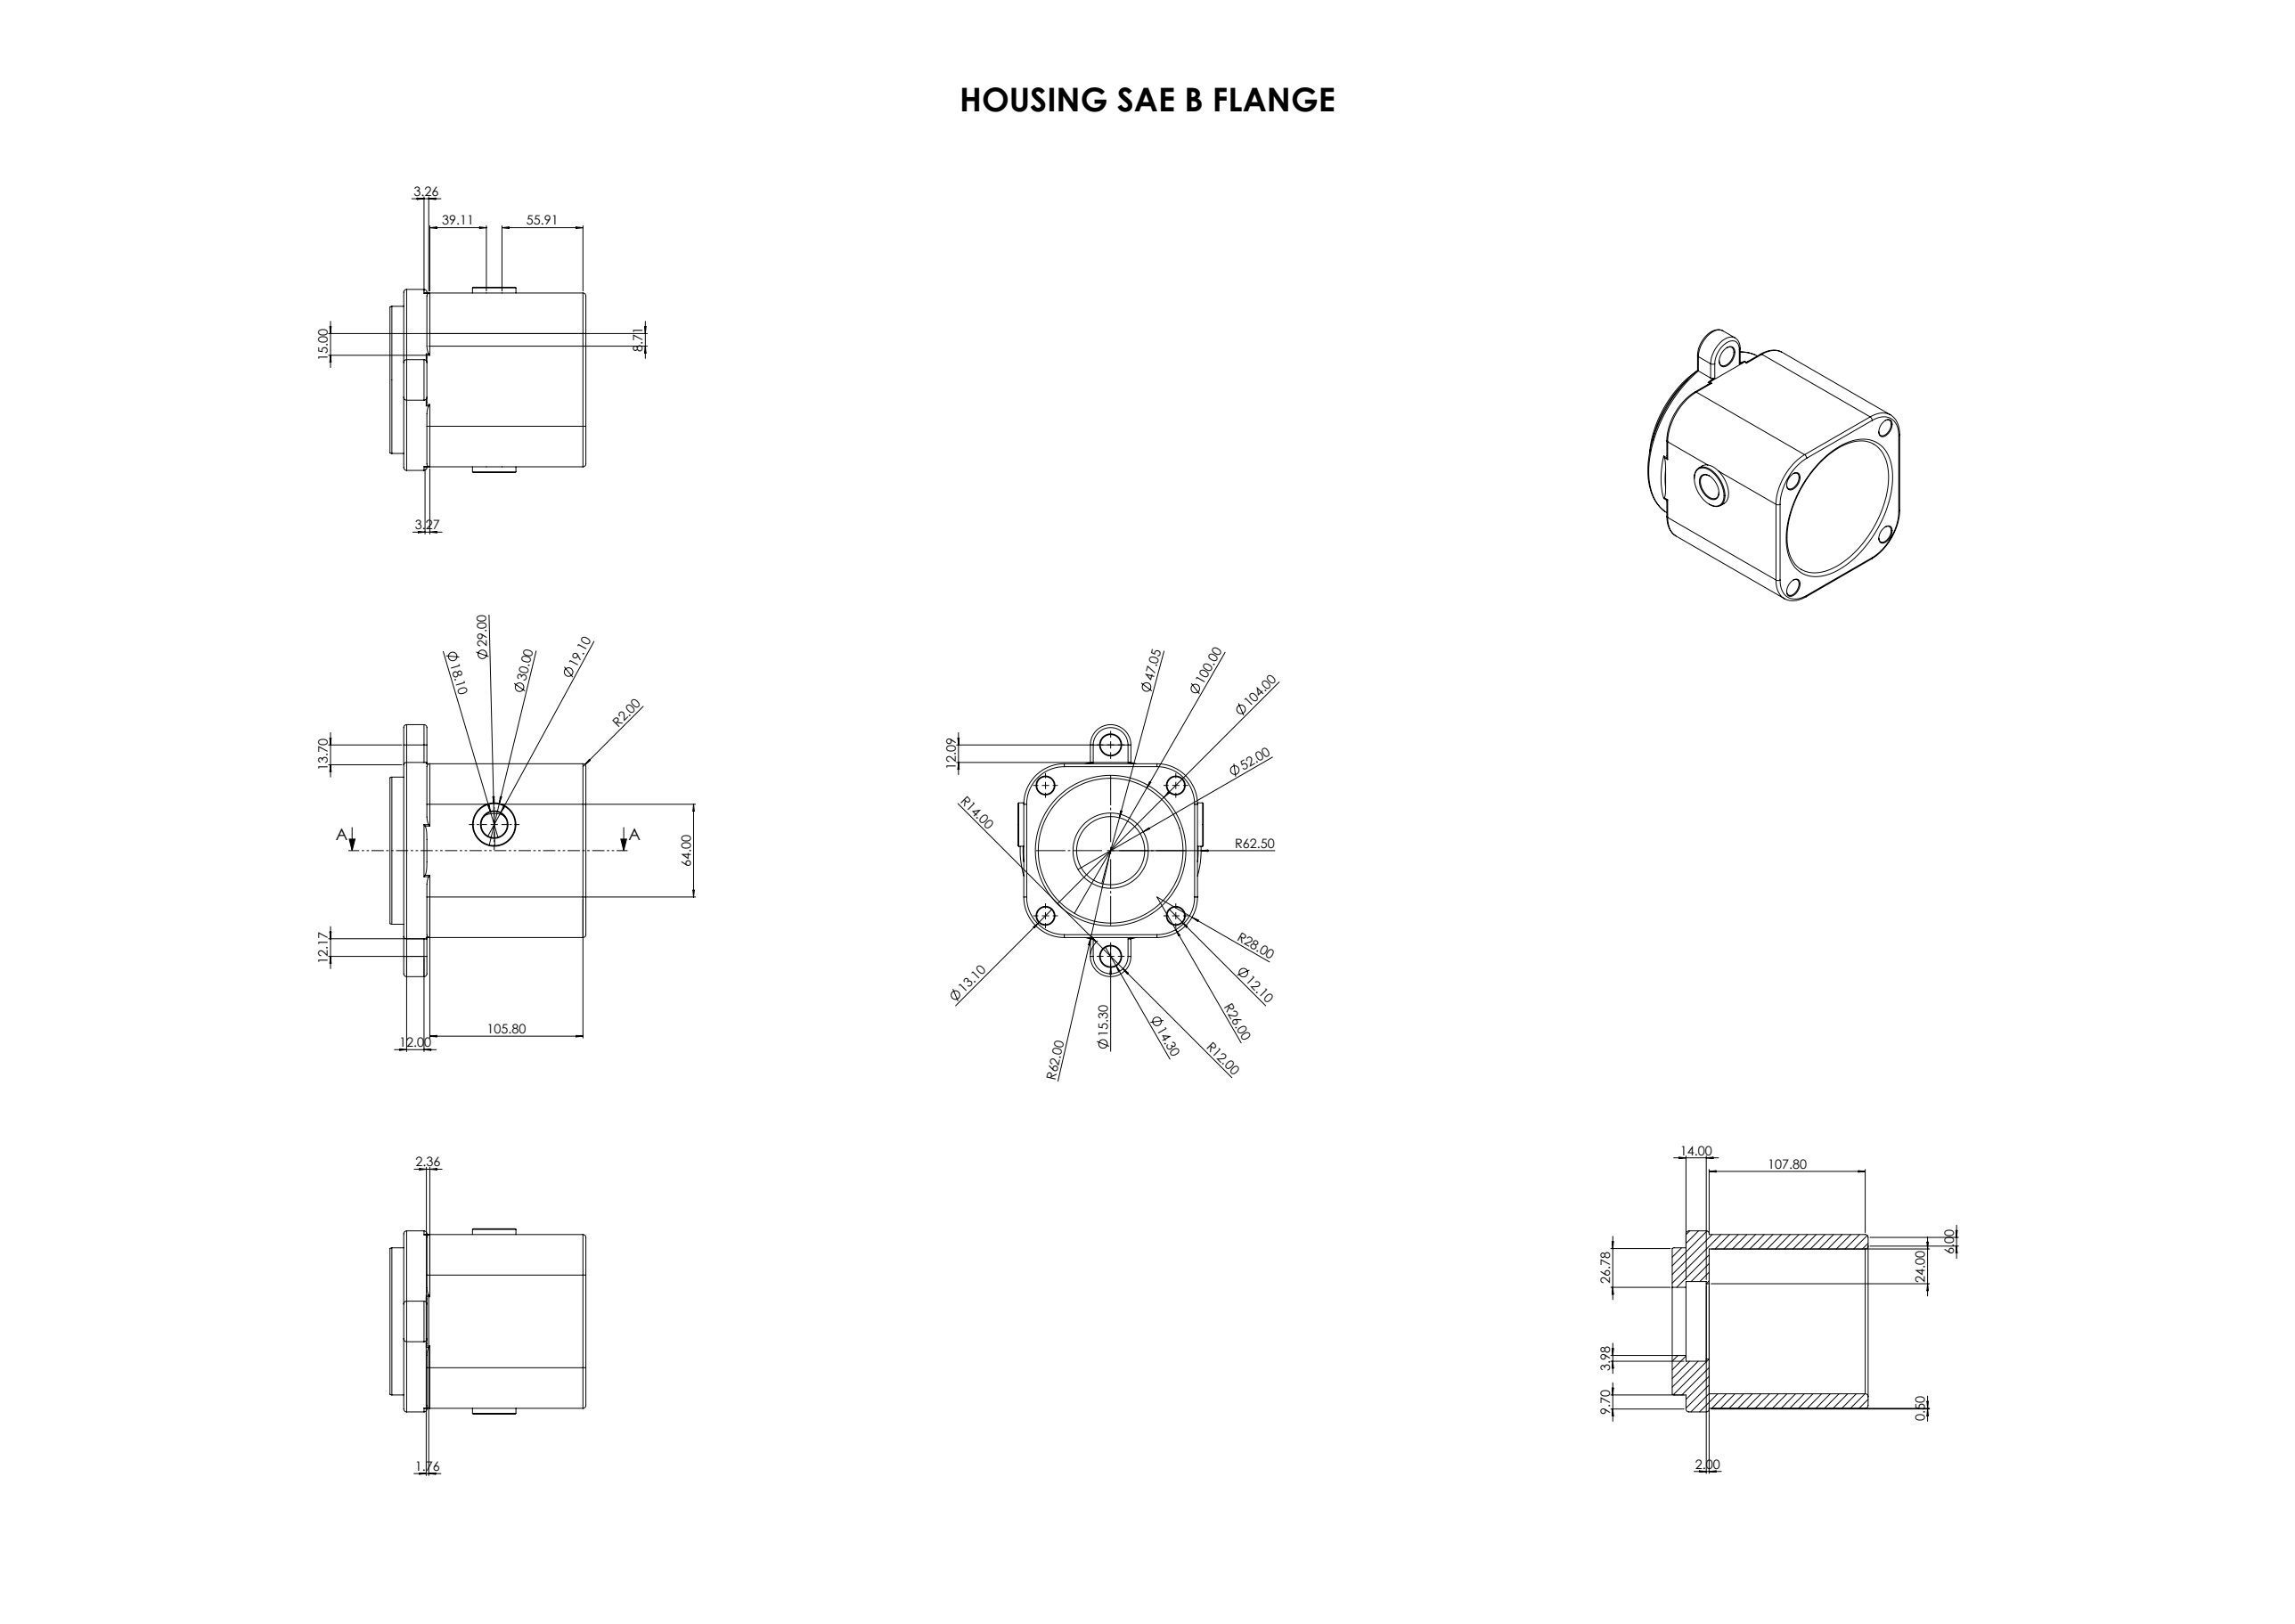
ISO-10303-21;
HEADER;
/* Generated by software containing ST-Developer
 * from STEP Tools, Inc. (www.steptools.com) 
 */

FILE_DESCRIPTION(
/* description */ (''),
/* implementation_level */ '2;1');

FILE_NAME(
/* name */ '01_Housing_SAE_B_Flange.step',
/* time_stamp */ '2026-10-26T07:49:00-07:00',
/* author */ (''),
/* organization */ (''),
/* preprocessor_version */ 'ST-DEVELOPER v20.2',
/* originating_system */ 'Autodesk Translation Framework v15.15.0.0',
/* authorisation */ '');

FILE_SCHEMA (('AUTOMOTIVE_DESIGN { 1 0 10303 214 3 1 1 }'));
ENDSEC;

DATA;
#10=MECHANICAL_DESIGN_GEOMETRIC_PRESENTATION_REPRESENTATION('',(#177),#38507);
#147=SHAPE_REPRESENTATION_RELATIONSHIP('SRR','None',#38575,#162);
#162=ADVANCED_BREP_SHAPE_REPRESENTATION('',(#192),#38492);
#177=STYLED_ITEM('',(#38699),#192);
#192=MANIFOLD_SOLID_BREP('Body1',#15071);
#207=B_SPLINE_SURFACE_WITH_KNOTS('',3,3,((#22067,#22068,#22069,#22070,#22071,
#22072,#22073),(#22074,#22075,#22076,#22077,#22078,#22079,#22080),(#22081,
#22082,#22083,#22084,#22085,#22086,#22087),(#22088,#22089,#22090,#22091,
#22092,#22093,#22094)),.UNSPECIFIED.,.F.,.F.,.F.,(4,4),(4,1,1,1,4),(0.,
1.),(-0.462000333519479,-0.263998422594088,-0.131997148643828,-0.0329961931811326,
4.1253064325321E-6),.UNSPECIFIED.);
#208=B_SPLINE_SURFACE_WITH_KNOTS('',3,3,((#22108,#22109,#22110,#22111,#22112,
#22113,#22114,#22115,#22116,#22117),(#22118,#22119,#22120,#22121,#22122,
#22123,#22124,#22125,#22126,#22127),(#22128,#22129,#22130,#22131,#22132,
#22133,#22134,#22135,#22136,#22137),(#22138,#22139,#22140,#22141,#22142,
#22143,#22144,#22145,#22146,#22147),(#22148,#22149,#22150,#22151,#22152,
#22153,#22154,#22155,#22156,#22157),(#22158,#22159,#22160,#22161,#22162,
#22163,#22164,#22165,#22166,#22167),(#22168,#22169,#22170,#22171,#22172,
#22173,#22174,#22175,#22176,#22177)),.UNSPECIFIED.,.F.,.F.,.F.,(4,1,1,1,
4),(4,1,1,1,1,1,1,4),(0.,0.285714285714286,0.571428571428571,0.785714285714286,
1.),(-7.35549329570849,-7.06046758790365,-6.76544188009881,-6.47041617229397,
-6.17539046448912,-5.88036475668429,-5.58533904887944,-5.2903133410746),
 .UNSPECIFIED.);
#209=B_SPLINE_SURFACE_WITH_KNOTS('',3,3,((#22179,#22180,#22181,#22182,#22183,
#22184,#22185,#22186,#22187,#22188,#22189,#22190,#22191,#22192,#22193,#22194,
#22195,#22196,#22197,#22198,#22199,#22200,#22201,#22202,#22203),(#22204,
#22205,#22206,#22207,#22208,#22209,#22210,#22211,#22212,#22213,#22214,#22215,
#22216,#22217,#22218,#22219,#22220,#22221,#22222,#22223,#22224,#22225,#22226,
#22227,#22228),(#22229,#22230,#22231,#22232,#22233,#22234,#22235,#22236,
#22237,#22238,#22239,#22240,#22241,#22242,#22243,#22244,#22245,#22246,#22247,
#22248,#22249,#22250,#22251,#22252,#22253),(#22254,#22255,#22256,#22257,
#22258,#22259,#22260,#22261,#22262,#22263,#22264,#22265,#22266,#22267,#22268,
#22269,#22270,#22271,#22272,#22273,#22274,#22275,#22276,#22277,#22278),
(#22279,#22280,#22281,#22282,#22283,#22284,#22285,#22286,#22287,#22288,
#22289,#22290,#22291,#22292,#22293,#22294,#22295,#22296,#22297,#22298,#22299,
#22300,#22301,#22302,#22303)),.UNSPECIFIED.,.F.,.F.,.F.,(4,1,4),(4,2,1,
1,1,1,1,1,1,1,1,1,1,1,1,1,1,1,1,1,1,4),(0.,0.571428571428571,1.),(-0.461724827521327,
-0.461389911948815,-0.455622538049454,-0.449855164150094,-0.438320416351374,
-0.415250920753933,-0.392181425156492,-0.369111929559052,-0.346042433961611,
-0.32297293836417,-0.29990344276673,-0.276833947169289,-0.253764451571848,
-0.230694955974407,-0.207625460376967,-0.196090712578246,-0.184555964779526,
-0.138416973584644,-0.115347477987204,-0.0922779823897629,-0.0461389911948815,
0.),.UNSPECIFIED.);
#210=B_SPLINE_SURFACE_WITH_KNOTS('',3,3,((#22314,#22315,#22316,#22317,#22318,
#22319,#22320,#22321,#22322,#22323),(#22324,#22325,#22326,#22327,#22328,
#22329,#22330,#22331,#22332,#22333),(#22334,#22335,#22336,#22337,#22338,
#22339,#22340,#22341,#22342,#22343),(#22344,#22345,#22346,#22347,#22348,
#22349,#22350,#22351,#22352,#22353),(#22354,#22355,#22356,#22357,#22358,
#22359,#22360,#22361,#22362,#22363),(#22364,#22365,#22366,#22367,#22368,
#22369,#22370,#22371,#22372,#22373)),.UNSPECIFIED.,.F.,.F.,.F.,(4,1,1,4),
(4,1,1,1,1,1,1,4),(0.,0.285714285714286,0.571428571428571,1.),(4.72327004783361,
5.43406096940559,6.14485189097757,6.85564281254955,7.56643373412153,8.27722465569351,
8.98801557726548,9.69880649883746),.UNSPECIFIED.);
#211=B_SPLINE_SURFACE_WITH_KNOTS('',3,3,((#22374,#22375,#22376,#22377,#22378,
#22379),(#22380,#22381,#22382,#22383,#22384,#22385),(#22386,#22387,#22388,
#22389,#22390,#22391),(#22392,#22393,#22394,#22395,#22396,#22397)),
 .UNSPECIFIED.,.F.,.F.,.F.,(4,4),(4,1,1,4),(0.,1.),(-0.461769339103211,
-0.197899101291517,-0.0659639823856703,3.57706725334641E-6),
 .UNSPECIFIED.);
#212=B_SPLINE_SURFACE_WITH_KNOTS('',3,3,((#22412,#22413,#22414,#22415,#22416,
#22417,#22418,#22419,#22420,#22421),(#22422,#22423,#22424,#22425,#22426,
#22427,#22428,#22429,#22430,#22431),(#22432,#22433,#22434,#22435,#22436,
#22437,#22438,#22439,#22440,#22441),(#22442,#22443,#22444,#22445,#22446,
#22447,#22448,#22449,#22450,#22451),(#22452,#22453,#22454,#22455,#22456,
#22457,#22458,#22459,#22460,#22461),(#22462,#22463,#22464,#22465,#22466,
#22467,#22468,#22469,#22470,#22471),(#22472,#22473,#22474,#22475,#22476,
#22477,#22478,#22479,#22480,#22481)),.UNSPECIFIED.,.F.,.F.,.F.,(4,1,1,1,
4),(4,1,1,1,1,1,1,4),(0.,0.285714285714286,0.571428571428571,0.785714285714286,
1.),(-7.35549329570849,-7.06046758790365,-6.76544188009881,-6.47041617229397,
-6.17539046448913,-5.88036475668429,-5.58533904887945,-5.29031334107461),
 .UNSPECIFIED.);
#213=B_SPLINE_SURFACE_WITH_KNOTS('',3,3,((#22485,#22486,#22487,#22488,#22489,
#22490),(#22491,#22492,#22493,#22494,#22495,#22496),(#22497,#22498,#22499,
#22500,#22501,#22502),(#22503,#22504,#22505,#22506,#22507,#22508)),
 .UNSPECIFIED.,.F.,.F.,.F.,(4,4),(4,1,1,4),(0.,1.),(-0.461725499841195,
-0.395764714149595,-0.263843142766397,0.),.UNSPECIFIED.);
#214=B_SPLINE_SURFACE_WITH_KNOTS('',3,3,((#22519,#22520,#22521,#22522,#22523,
#22524,#22525,#22526,#22527,#22528),(#22529,#22530,#22531,#22532,#22533,
#22534,#22535,#22536,#22537,#22538),(#22539,#22540,#22541,#22542,#22543,
#22544,#22545,#22546,#22547,#22548),(#22549,#22550,#22551,#22552,#22553,
#22554,#22555,#22556,#22557,#22558),(#22559,#22560,#22561,#22562,#22563,
#22564,#22565,#22566,#22567,#22568),(#22569,#22570,#22571,#22572,#22573,
#22574,#22575,#22576,#22577,#22578)),.UNSPECIFIED.,.F.,.F.,.F.,(4,1,1,4),
(4,1,1,1,1,1,1,4),(0.,0.285714285714286,0.571428571428571,1.),(4.72327004804774,
5.43406096961972,6.1448518911917,6.85564281276368,7.56643373433566,8.27722465590764,
8.98801557747962,9.6988064990516),.UNSPECIFIED.);
#256=TOROIDAL_SURFACE('',#15366,60.5,2.);
#257=TOROIDAL_SURFACE('',#15369,12.,2.);
#258=TOROIDAL_SURFACE('',#15373,60.5,2.);
#259=TOROIDAL_SURFACE('',#15374,12.,2.);
#260=TOROIDAL_SURFACE('',#15383,60.5,2.);
#261=TOROIDAL_SURFACE('',#15387,12.,2.);
#262=TOROIDAL_SURFACE('',#15394,60.5,2.);
#263=TOROIDAL_SURFACE('',#15398,12.,2.);
#264=TOROIDAL_SURFACE('',#15402,48.8,2.);
#265=TOROIDAL_SURFACE('',#15409,26.,2.);
#266=TOROIDAL_SURFACE('',#15415,26.,2.);
#267=TOROIDAL_SURFACE('',#15425,26.,2.);
#268=TOROIDAL_SURFACE('',#15433,26.,2.);
#269=TOROIDAL_SURFACE('',#15442,26.,2.);
#270=TOROIDAL_SURFACE('',#15447,26.,2.);
#271=TOROIDAL_SURFACE('',#15452,26.,2.);
#272=TOROIDAL_SURFACE('',#15457,26.,2.);
#273=TOROIDAL_SURFACE('',#15461,52.,2.);
#293=ELLIPSE('',#15321,13.946906437048,2.);
#294=ELLIPSE('',#15324,13.946906437048,2.);
#295=ELLIPSE('',#15327,13.946906437048,2.);
#296=ELLIPSE('',#15331,13.946906437048,2.);
#297=ELLIPSE('',#15340,13.946906437048,2.);
#298=ELLIPSE('',#15343,13.946906437048,2.);
#299=ELLIPSE('',#15346,13.946906437048,2.);
#300=ELLIPSE('',#15350,13.946906437048,2.);
#332=(
BOUNDED_CURVE()
B_SPLINE_CURVE(2,(#21090,#21091,#21092),.UNSPECIFIED.,.F.,.F.)
B_SPLINE_CURVE_WITH_KNOTS((3,3),(-9.16934047811363,-8.99429341935052),
 .UNSPECIFIED.)
CURVE()
GEOMETRIC_REPRESENTATION_ITEM()
RATIONAL_B_SPLINE_CURVE((1.20544110146931,1.20730170334354,1.20901639344262))
REPRESENTATION_ITEM('')
);
#333=(
BOUNDED_CURVE()
B_SPLINE_CURVE(2,(#21112,#21113,#21114),.UNSPECIFIED.,.F.,.F.)
B_SPLINE_CURVE_WITH_KNOTS((3,3),(-4.88014350616112,-4.705096447398),
 .UNSPECIFIED.)
CURVE()
GEOMETRIC_REPRESENTATION_ITEM()
RATIONAL_B_SPLINE_CURVE((1.20901639344263,1.20730170334354,1.20544110146931))
REPRESENTATION_ITEM('')
);
#334=(
BOUNDED_CURVE()
B_SPLINE_CURVE(2,(#21198,#21199,#21200),.UNSPECIFIED.,.F.,.F.)
B_SPLINE_CURVE_WITH_KNOTS((3,3),(-4.88014350616107,-4.70509644739795),
 .UNSPECIFIED.)
CURVE()
GEOMETRIC_REPRESENTATION_ITEM()
RATIONAL_B_SPLINE_CURVE((1.20901639344262,1.20730170334354,1.20544110146931))
REPRESENTATION_ITEM('')
);
#335=(
BOUNDED_CURVE()
B_SPLINE_CURVE(2,(#21291,#21292,#21293),.UNSPECIFIED.,.F.,.F.)
B_SPLINE_CURVE_WITH_KNOTS((3,3),(-9.16934047811369,-8.99429341935056),
 .UNSPECIFIED.)
CURVE()
GEOMETRIC_REPRESENTATION_ITEM()
RATIONAL_B_SPLINE_CURVE((1.20544110146931,1.20730170334354,1.20901639344263))
REPRESENTATION_ITEM('')
);
#417=FACE_BOUND('',#2507,.T.);
#418=FACE_BOUND('',#2510,.T.);
#419=FACE_BOUND('',#2514,.T.);
#420=FACE_BOUND('',#2518,.T.);
#421=FACE_BOUND('',#2524,.T.);
#422=FACE_BOUND('',#2525,.T.);
#423=FACE_BOUND('',#2526,.T.);
#424=FACE_BOUND('',#2527,.T.);
#425=FACE_BOUND('',#2528,.T.);
#426=FACE_BOUND('',#2556,.T.);
#427=FACE_BOUND('',#2557,.T.);
#428=FACE_BOUND('',#2558,.T.);
#429=FACE_BOUND('',#2612,.T.);
#430=FACE_BOUND('',#2613,.T.);
#431=FACE_BOUND('',#2629,.T.);
#432=FACE_BOUND('',#2632,.T.);
#433=FACE_BOUND('',#2635,.T.);
#434=FACE_BOUND('',#2637,.T.);
#558=PLANE('',#15260);
#559=PLANE('',#15265);
#560=PLANE('',#15274);
#561=PLANE('',#15282);
#562=PLANE('',#15295);
#563=PLANE('',#15320);
#564=PLANE('',#15322);
#565=PLANE('',#15323);
#566=PLANE('',#15325);
#567=PLANE('',#15326);
#568=PLANE('',#15330);
#569=PLANE('',#15339);
#570=PLANE('',#15341);
#571=PLANE('',#15342);
#572=PLANE('',#15344);
#573=PLANE('',#15345);
#574=PLANE('',#15349);
#575=PLANE('',#15358);
#576=PLANE('',#15382);
#577=PLANE('',#15391);
#578=PLANE('',#15393);
#579=PLANE('',#15401);
#580=PLANE('',#15414);
#581=PLANE('',#15422);
#582=PLANE('',#15430);
#583=PLANE('',#15438);
#584=PLANE('',#15473);
#585=PLANE('',#15474);
#586=PLANE('',#15475);
#587=PLANE('',#15476);
#588=PLANE('',#15480);
#589=PLANE('',#15484);
#590=PLANE('',#15488);
#591=PLANE('',#15489);
#592=PLANE('',#15492);
#593=PLANE('',#15493);
#1009=B_SPLINE_CURVE_WITH_KNOTS('',3,(#20904,#20905,#20906,#20907,#20908,
#20909,#20910,#20911,#20912,#20913),.UNSPECIFIED.,.F.,.F.,(4,2,2,2,4),(3.93196561503714,
3.98793494995107,4.45544073881652,4.92294652768197,4.9789158625959),
 .UNSPECIFIED.);
#1010=B_SPLINE_CURVE_WITH_KNOTS('',3,(#20956,#20957,#20958,#20959,#20960,
#20961,#20962,#20963,#20964,#20965),.UNSPECIFIED.,.F.,.F.,(4,2,2,2,4),(3.93196561503714,
3.98793494995108,4.45544073881652,4.92294652768197,4.97891586259591),
 .UNSPECIFIED.);
#1011=B_SPLINE_CURVE_WITH_KNOTS('',3,(#20998,#20999,#21000,#21001,#21002),
 .UNSPECIFIED.,.F.,.F.,(4,1,4),(4.72327004821084,5.43406096940559,5.4438775737049),
 .UNSPECIFIED.);
#1012=B_SPLINE_CURVE_WITH_KNOTS('',3,(#21005,#21006,#21007,#21008,#21009,
#21010,#21011,#21012,#21013),.UNSPECIFIED.,.F.,.F.,(4,1,1,1,1,1,4),(5.4438775737049,
6.14485189097757,6.85564281254955,7.56643373412153,8.27722465569351,8.98801557726548,
9.69880649883746),.UNSPECIFIED.);
#1013=B_SPLINE_CURVE_WITH_KNOTS('',3,(#21075,#21076,#21077,#21078,#21079,
#21080,#21081,#21082),.UNSPECIFIED.,.F.,.F.,(4,2,2,4),(0.909514729117648,
0.949358494570548,1.0210248366573,1.05494162626089),.UNSPECIFIED.);
#1014=B_SPLINE_CURVE_WITH_KNOTS('',3,(#21086,#21087,#21088,#21089),
 .UNSPECIFIED.,.F.,.F.,(4,4),(-0.0999299837778113,0.),.UNSPECIFIED.);
#1015=B_SPLINE_CURVE_WITH_KNOTS('',3,(#21118,#21119,#21120,#21121,#21122,
#21123,#21124,#21125,#21126,#21127),.UNSPECIFIED.,.F.,.F.,(4,2,2,2,4),(2.62788407869953,
2.67944373713314,2.73012587368336,2.74303185768817,2.7532959630073),
 .UNSPECIFIED.);
#1016=B_SPLINE_CURVE_WITH_KNOTS('',3,(#21137,#21138,#21139,#21140,#21141,
#21142,#21143,#21144,#21145,#21146),.UNSPECIFIED.,.F.,.F.,(4,2,2,2,4),(1.79948460602208,
1.8527312039325,2.06373263634258,2.27473406875267,2.69673693357283),
 .UNSPECIFIED.);
#1017=B_SPLINE_CURVE_WITH_KNOTS('',3,(#21150,#21151,#21152,#21153,#21154,
#21155,#21156,#21157,#21158,#21159),.UNSPECIFIED.,.F.,.F.,(4,2,2,2,4),(4.15220051801173,
4.5742033828319,4.78520481524198,4.99620624765207,5.04945284556248),
 .UNSPECIFIED.);
#1018=B_SPLINE_CURVE_WITH_KNOTS('',3,(#21174,#21175,#21176,#21177,#21178,
#21179,#21180,#21181,#21182,#21183),.UNSPECIFIED.,.F.,.F.,(4,2,2,2,4),(0.917765321002435,
0.928029426321564,0.940935410326375,0.991617546876601,1.04317720531021),
 .UNSPECIFIED.);
#1019=B_SPLINE_CURVE_WITH_KNOTS('',3,(#21189,#21190,#21191,#21192,#21193,
#21194,#21195,#21196),.UNSPECIFIED.,.F.,.F.,(4,2,2,4),(0.423927454431935,
0.457844244035524,0.529510586122272,0.569354351575173),.UNSPECIFIED.);
#1020=B_SPLINE_CURVE_WITH_KNOTS('',3,(#21201,#21202,#21203,#21204),
 .UNSPECIFIED.,.F.,.F.,(4,4),(-0.0999299524181728,0.),.UNSPECIFIED.);
#1021=B_SPLINE_CURVE_WITH_KNOTS('',3,(#21213,#21214,#21215,#21216,#21217,
#21218,#21219,#21220),.UNSPECIFIED.,.F.,.F.,(4,2,2,4),(0.444478348171076,
0.457897885991393,0.533188282866212,0.608478679741031),.UNSPECIFIED.);
#1022=B_SPLINE_CURVE_WITH_KNOTS('',3,(#21227,#21228,#21229,#21230,#21231,
#21232,#21233,#21234),.UNSPECIFIED.,.F.,.F.,(4,2,2,4),(0.608478679741031,
0.68376907661585,0.759059473490669,0.772479011310987),.UNSPECIFIED.);
#1023=B_SPLINE_CURVE_WITH_KNOTS('',3,(#21236,#21237,#21238,#21239,#21240,
#21241,#21242,#21243),.UNSPECIFIED.,.F.,.F.,(4,2,2,4),(1.27628724021533,
1.34251720334849,1.43059045082634,1.8254794159769),.UNSPECIFIED.);
#1024=B_SPLINE_CURVE_WITH_KNOTS('',3,(#21246,#21247,#21248,#21249,#21250,
#21251,#21252,#21253),.UNSPECIFIED.,.F.,.F.,(4,2,2,4),(0.537818085774576,
0.932707050925141,1.02078029840299,1.08701026153615),.UNSPECIFIED.);
#1025=B_SPLINE_CURVE_WITH_KNOTS('',3,(#21256,#21257,#21258,#21259,#21260,
#21261,#21262,#21263),.UNSPECIFIED.,.F.,.F.,(4,2,2,4),(1.27628724021533,
1.34251720334849,1.43059045082634,1.8254794159769),.UNSPECIFIED.);
#1026=B_SPLINE_CURVE_WITH_KNOTS('',3,(#21266,#21267,#21268,#21269,#21270,
#21271,#21272,#21273),.UNSPECIFIED.,.F.,.F.,(4,2,2,4),(0.537818085774576,
0.932707050925141,1.02078029840299,1.08701026153615),.UNSPECIFIED.);
#1027=B_SPLINE_CURVE_WITH_KNOTS('',3,(#21276,#21277,#21278,#21279,#21280,
#21281,#21282,#21283),.UNSPECIFIED.,.F.,.F.,(4,2,2,4),(0.909514729117652,
0.949358494570554,1.0210248366573,1.05494162626089),.UNSPECIFIED.);
#1028=B_SPLINE_CURVE_WITH_KNOTS('',3,(#21287,#21288,#21289,#21290),
 .UNSPECIFIED.,.F.,.F.,(4,4),(-0.099929983777859,0.),.UNSPECIFIED.);
#1029=B_SPLINE_CURVE_WITH_KNOTS('',3,(#21313,#21314,#21315,#21316,#21317,
#21318,#21319,#21320,#21321,#21322),.UNSPECIFIED.,.F.,.F.,(4,2,2,2,4),(2.62788407869953,
2.67944373713314,2.73012587368336,2.74303185768817,2.7532959630073),
 .UNSPECIFIED.);
#1030=B_SPLINE_CURVE_WITH_KNOTS('',3,(#21332,#21333,#21334,#21335,#21336,
#21337,#21338,#21339,#21340,#21341),.UNSPECIFIED.,.F.,.F.,(4,2,2,2,4),(1.79948460602208,
1.8527312039325,2.06373263634258,2.27473406875267,2.69673693357283),
 .UNSPECIFIED.);
#1031=B_SPLINE_CURVE_WITH_KNOTS('',3,(#21345,#21346,#21347,#21348,#21349,
#21350,#21351,#21352,#21353,#21354),.UNSPECIFIED.,.F.,.F.,(4,2,2,2,4),(4.15220051801173,
4.5742033828319,4.78520481524198,4.99620624765207,5.04945284556248),
 .UNSPECIFIED.);
#1032=B_SPLINE_CURVE_WITH_KNOTS('',3,(#21369,#21370,#21371,#21372,#21373,
#21374,#21375,#21376,#21377,#21378),.UNSPECIFIED.,.F.,.F.,(4,2,2,2,4),(0.917765321002435,
0.928029426321564,0.940935410326375,0.991617546876601,1.04317720531021),
 .UNSPECIFIED.);
#1033=B_SPLINE_CURVE_WITH_KNOTS('',3,(#21384,#21385,#21386,#21387,#21388,
#21389,#21390,#21391),.UNSPECIFIED.,.F.,.F.,(4,2,2,4),(0.42392745443194,
0.457844244035527,0.529510586122276,0.569354351575178),.UNSPECIFIED.);
#1034=B_SPLINE_CURVE_WITH_KNOTS('',3,(#21392,#21393,#21394,#21395),
 .UNSPECIFIED.,.F.,.F.,(4,4),(-0.0999299524180764,0.),.UNSPECIFIED.);
#1035=B_SPLINE_CURVE_WITH_KNOTS('',3,(#21402,#21403,#21404,#21405,#21406,
#21407,#21408,#21409),.UNSPECIFIED.,.F.,.F.,(4,2,2,4),(0.444478348171076,
0.457897885991393,0.533188282866212,0.608478679741031),.UNSPECIFIED.);
#1036=B_SPLINE_CURVE_WITH_KNOTS('',3,(#21416,#21417,#21418,#21419,#21420,
#21421,#21422,#21423),.UNSPECIFIED.,.F.,.F.,(4,2,2,4),(0.608478679741031,
0.68376907661585,0.759059473490669,0.772479011310987),.UNSPECIFIED.);
#1037=B_SPLINE_CURVE_WITH_KNOTS('',3,(#21425,#21426,#21427,#21428,#21429,
#21430,#21431,#21432),.UNSPECIFIED.,.F.,.F.,(4,2,2,4),(1.27628724021533,
1.34251720334849,1.43059045082634,1.8254794159769),.UNSPECIFIED.);
#1038=B_SPLINE_CURVE_WITH_KNOTS('',3,(#21435,#21436,#21437,#21438,#21439,
#21440,#21441,#21442),.UNSPECIFIED.,.F.,.F.,(4,2,2,4),(0.537818085774576,
0.932707050925141,1.02078029840299,1.08701026153615),.UNSPECIFIED.);
#1039=B_SPLINE_CURVE_WITH_KNOTS('',3,(#21445,#21446,#21447,#21448,#21449,
#21450,#21451,#21452),.UNSPECIFIED.,.F.,.F.,(4,2,2,4),(1.27628724021533,
1.34251720334849,1.43059045082634,1.8254794159769),.UNSPECIFIED.);
#1040=B_SPLINE_CURVE_WITH_KNOTS('',3,(#21455,#21456,#21457,#21458,#21459,
#21460,#21461,#21462),.UNSPECIFIED.,.F.,.F.,(4,2,2,4),(0.537818085774576,
0.932707050925141,1.02078029840299,1.08701026153615),.UNSPECIFIED.);
#1041=B_SPLINE_CURVE_WITH_KNOTS('',3,(#21491,#21492,#21493,#21494,#21495,
#21496,#21497,#21498,#21499,#21500,#21501,#21502,#21503,#21504),
 .UNSPECIFIED.,.F.,.F.,(4,2,2,2,2,2,4),(-0.0007960460749726,0.,0.0734612670102269,
0.144831741121295,0.230214082122091,0.299049896049864,0.361337990313849),
 .UNSPECIFIED.);
#1042=B_SPLINE_CURVE_WITH_KNOTS('',3,(#21505,#21506,#21507,#21508,#21509,
#21510,#21511,#21512,#21513,#21514,#21515,#21516,#21517,#21518),
 .UNSPECIFIED.,.F.,.F.,(4,2,2,2,2,2,4),(-0.723464285927595,-0.722647521542398,
-0.649394023974264,-0.578539147977434,-0.492689132311904,-0.42364974758642,
-0.361323760770171),.UNSPECIFIED.);
#1043=B_SPLINE_CURVE_WITH_KNOTS('',3,(#21528,#21529,#21530,#21531,#21532,
#21533,#21534,#21535,#21536,#21537,#21538,#21539,#21540,#21541),
 .UNSPECIFIED.,.F.,.F.,(4,2,2,2,2,2,4),(-0.361281373349619,-0.299845297677646,
-0.234790847494551,-0.156277186792366,-0.0770809532846638,0.,0.000773217160646022),
 .UNSPECIFIED.);
#1044=B_SPLINE_CURVE_WITH_KNOTS('',3,(#21544,#21545,#21546,#21547,#21548,
#21549,#21550,#21551,#21552,#21553,#21554,#21555,#21556,#21557),
 .UNSPECIFIED.,.F.,.F.,(4,2,2,2,2,2,4),(-0.723464285923361,-0.722647521538168,
-0.649394023970219,-0.578539147973825,-0.492689132308839,-0.423649747583786,
-0.361323760767944),.UNSPECIFIED.);
#1045=B_SPLINE_CURVE_WITH_KNOTS('',3,(#21692,#21693,#21694,#21695,#21696,
#21697,#21698,#21699,#21700,#21701,#21702,#21703,#21704,#21705,#21706,#21707,
#21708,#21709,#21710,#21711,#21712,#21713,#21714,#21715,#21716),
 .UNSPECIFIED.,.F.,.F.,(4,1,1,1,1,1,1,1,1,1,1,1,1,1,1,1,1,1,1,1,2,4),(0.,
0.0461389911948815,0.0922779823897629,0.115347477987204,0.138416973584644,
0.184555964779526,0.196090712578246,0.207625460376967,0.230694955974407,
0.253764451571848,0.276833947169289,0.29990344276673,0.32297293836417,0.346042433961611,
0.369111929559052,0.392181425156492,0.415250920753933,0.438320416351374,
0.449855164150094,0.455622538049454,0.461389911948815,0.46172446147336),
 .UNSPECIFIED.);
#1046=B_SPLINE_CURVE_WITH_KNOTS('',3,(#21718,#21719,#21720,#21721,#21722,
#21723,#21724,#21725,#21726,#21727),.UNSPECIFIED.,.F.,.F.,(4,1,1,1,1,1,
1,4),(5.2903133410746,5.58533904887944,5.88036475668429,6.17539046448912,
6.47041617229397,6.76544188009881,7.06046758790365,7.35549329570849),
 .UNSPECIFIED.);
#1047=B_SPLINE_CURVE_WITH_KNOTS('',3,(#21729,#21730,#21731,#21732,#21733,
#21734,#21735),.UNSPECIFIED.,.F.,.F.,(4,1,1,1,4),(-4.1253064325321E-6,0.0329961931811326,
0.131997148643828,0.263998422594088,0.462000333519479),.UNSPECIFIED.);
#1048=B_SPLINE_CURVE_WITH_KNOTS('',3,(#21736,#21737,#21738,#21739,#21740,
#21741,#21742,#21743,#21744,#21745,#21746,#21747,#21748,#21749,#21750,#21751,
#21752,#21753,#21754,#21755,#21756,#21757,#21758,#21759,#21760,#21761,#21762,
#21763,#21764,#21765,#21766,#21767,#21768,#21769,#21770,#21771,#21772,#21773,
#21774,#21775,#21776,#21777,#21778,#21779,#21780,#21781,#21782,#21783,#21784,
#21785,#21786,#21787,#21788,#21789,#21790,#21791,#21792,#21793,#21794,#21795,
#21796,#21797,#21798,#21799,#21800,#21801,#21802,#21803,#21804,#21805,#21806,
#21807,#21808,#21809,#21810,#21811,#21812,#21813,#21814,#21815,#21816,#21817,
#21818,#21819,#21820,#21821,#21822,#21823,#21824,#21825,#21826,#21827,#21828,
#21829,#21830,#21831,#21832,#21833,#21834,#21835,#21836,#21837,#21838,#21839,
#21840,#21841,#21842,#21843,#21844,#21845,#21846,#21847,#21848,#21849,#21850,
#21851,#21852,#21853,#21854,#21855,#21856,#21857,#21858,#21859,#21860,#21861,
#21862,#21863,#21864,#21865,#21866,#21867,#21868,#21869,#21870,#21871,#21872,
#21873,#21874,#21875,#21876,#21877,#21878,#21879,#21880,#21881,#21882,#21883,
#21884,#21885,#21886,#21887,#21888,#21889),.UNSPECIFIED.,.F.,.F.,(4,3,3,
3,3,3,3,3,3,3,3,3,3,3,3,3,3,3,3,3,3,3,3,3,3,3,3,3,3,3,3,3,3,3,3,3,3,3,3,
3,3,3,3,3,3,3,3,3,3,3,3,4),(-9.23633566839803,-9.12960054610899,-9.02995313475932,
-8.98820092273608,-8.94767164911647,-8.85551547280586,-8.76973813956101,
-8.76335929649525,-8.67204037852948,-8.58170123880419,-8.50986230805487,
-8.41197083977331,-8.31595106965646,-8.27742304064402,-8.18141772850045,
-8.08522998019979,-8.07506594002406,-7.96624383986804,-7.85665330525787,
-7.74811076545733,-7.64783984054416,-7.56639692453424,-7.46050702505756,
-7.35408928718672,-7.24751062386446,-7.21105298394138,-7.11797817184964,
-7.02480289993274,-6.98739369316414,-6.87981578778465,-6.85563657893624,
-6.75528006343046,-6.64913220023725,-6.54164653415872,-6.43390512945243,
-6.37349276133023,-6.27658287658477,-6.1795448081392,-6.14462846979886,
-6.04725880022175,-5.9475667529657,-5.93469080516676,-5.83694309104053,
-5.73794849627641,-5.67251567403569,-5.57655253596878,-5.48609949444031,
-5.43374272495868,-5.34284104121183,-5.3056567205391,-5.19777701987056,
-5.18574149361684),.UNSPECIFIED.);
#1049=B_SPLINE_CURVE_WITH_KNOTS('',3,(#21892,#21893,#21894,#21895,#21896,
#21897),.UNSPECIFIED.,.F.,.F.,(4,1,1,4),(0.,0.263843142766397,0.395764714149595,
0.461725499841195),.UNSPECIFIED.);
#1050=B_SPLINE_CURVE_WITH_KNOTS('',3,(#21899,#21900,#21901,#21902,#21903,
#21904,#21905,#21906,#21907,#21908),.UNSPECIFIED.,.F.,.F.,(4,1,1,1,1,1,
1,4),(5.29031334107461,5.58533904887945,5.88036475668429,6.17539046448913,
6.47041617229397,6.76544188009881,7.06046758790365,7.35549329570849),
 .UNSPECIFIED.);
#1051=B_SPLINE_CURVE_WITH_KNOTS('',3,(#21910,#21911,#21912,#21913,#21914,
#21915),.UNSPECIFIED.,.F.,.F.,(4,1,1,4),(-3.57706725334641E-6,0.0659639823856703,
0.197899101291517,0.461769339103211),.UNSPECIFIED.);
#1052=B_SPLINE_CURVE_WITH_KNOTS('',3,(#21916,#21917,#21918,#21919,#21920,
#21921,#21922,#21923,#21924,#21925,#21926,#21927,#21928,#21929,#21930,#21931,
#21932,#21933,#21934,#21935,#21936,#21937,#21938,#21939,#21940,#21941,#21942,
#21943,#21944,#21945,#21946,#21947,#21948,#21949,#21950,#21951,#21952,#21953,
#21954,#21955,#21956,#21957,#21958,#21959,#21960,#21961,#21962,#21963,#21964,
#21965,#21966,#21967,#21968,#21969,#21970,#21971,#21972,#21973,#21974,#21975,
#21976,#21977,#21978,#21979,#21980,#21981,#21982,#21983,#21984,#21985,#21986,
#21987,#21988,#21989,#21990,#21991,#21992,#21993,#21994,#21995,#21996,#21997,
#21998,#21999,#22000,#22001,#22002,#22003,#22004,#22005,#22006,#22007,#22008,
#22009,#22010,#22011,#22012,#22013,#22014,#22015,#22016,#22017,#22018,#22019,
#22020,#22021,#22022,#22023,#22024,#22025,#22026,#22027,#22028,#22029,#22030,
#22031,#22032,#22033,#22034,#22035,#22036,#22037,#22038,#22039,#22040,#22041,
#22042,#22043,#22044,#22045,#22046,#22047,#22048,#22049,#22050,#22051,#22052,
#22053,#22054,#22055,#22056,#22057,#22058,#22059,#22060,#22061,#22062,#22063,
#22064,#22065,#22066),.UNSPECIFIED.,.F.,.F.,(4,3,3,3,3,3,3,3,3,3,3,3,3,
3,3,3,3,3,3,3,3,3,3,3,3,3,3,3,3,3,3,3,3,3,3,3,3,3,3,3,3,3,3,3,3,3,3,3,3,
3,4),(-9.23633566861216,-9.12960054616757,-9.0301001347754,-8.98819964439314,
-8.9476716491939,-8.85551547287179,-8.77004832787379,-8.76335929654967,
-8.67183742403758,-8.58130233357639,-8.50986230801197,-8.41188984789292,
-8.31575746142269,-8.277426795238,-8.17624636762553,-8.07506594001306,-7.96541085300417,
-7.85497781952315,-7.74563908368099,-7.64783984052849,-7.56643652217298,
-7.46139284189079,-7.35584564549624,-7.25012317373638,-7.21105298394139,
-7.1181354465781,-7.02511356178625,-6.98739369309937,-6.88169773695743,
-6.85571344061752,-6.75528006328435,-6.64904197167172,-6.54161818053077,
-6.43368025611171,-6.37349276120329,-6.27597952064751,-6.17860698749197,
-6.14486393337072,-6.04674431800307,-5.94656644708164,-5.93469080503813,
-5.83307322116587,-5.7296525497896,-5.67251567404192,-5.56269437350081,
-5.48609949447997,-5.43365613366603,-5.33247743921033,-5.30565672055846,
-5.20312542921902,-5.18574149383096),.UNSPECIFIED.);
#1053=B_SPLINE_CURVE_WITH_KNOTS('',3,(#22096,#22097,#22098,#22099,#22100,
#22101,#22102,#22103,#22104,#22105,#22106,#22107),.UNSPECIFIED.,.F.,.F.,
(4,2,2,2,2,4),(0.,0.374578330850399,0.631956342435387,0.751788955793774,
0.804327350058264,0.853099247911436),.UNSPECIFIED.);
#1054=B_SPLINE_CURVE_WITH_KNOTS('',3,(#22304,#22305,#22306,#22307,#22308,
#22309,#22310,#22311,#22312,#22313),.UNSPECIFIED.,.F.,.F.,(4,2,2,2,4),(0.,
0.0337361869540046,0.0857366303783598,0.186224664796239,0.342354568854618),
 .UNSPECIFIED.);
#1055=B_SPLINE_CURVE_WITH_KNOTS('',3,(#22400,#22401,#22402,#22403,#22404,
#22405,#22406,#22407,#22408,#22409,#22410,#22411),.UNSPECIFIED.,.F.,.F.,
(4,2,2,2,2,4),(0.,0.374578330850087,0.63195634243358,0.751788955791072,
0.804327350055048,0.853099247907485),.UNSPECIFIED.);
#1056=B_SPLINE_CURVE_WITH_KNOTS('',3,(#22509,#22510,#22511,#22512,#22513,
#22514,#22515,#22516,#22517,#22518),.UNSPECIFIED.,.F.,.F.,(4,3,3,4),(0.,
0.0489077955509596,0.146723386652879,0.342354568856692),.UNSPECIFIED.);
#1057=B_SPLINE_CURVE_WITH_KNOTS('',3,(#22580,#22581,#22582,#22583,#22584,
#22585,#22586,#22587,#22588),.UNSPECIFIED.,.F.,.F.,(4,1,1,1,1,1,4),(4.72327004842498,
5.43406096961972,6.1448518911917,6.85564281276368,7.56643373433566,8.27722465590764,
8.97833931241972),.UNSPECIFIED.);
#1058=B_SPLINE_CURVE_WITH_KNOTS('',3,(#22589,#22590,#22591,#22592,#22593),
 .UNSPECIFIED.,.F.,.F.,(4,1,4),(8.97833931241972,8.98801557747962,9.6988064990516),
 .UNSPECIFIED.);
#1366=CYLINDRICAL_SURFACE('',#15257,15.);
#1367=CYLINDRICAL_SURFACE('',#15269,7.15);
#1368=CYLINDRICAL_SURFACE('',#15276,15.);
#1369=CYLINDRICAL_SURFACE('',#15286,7.15);
#1370=CYLINDRICAL_SURFACE('',#15290,9.05);
#1371=CYLINDRICAL_SURFACE('',#15304,6.05);
#1372=CYLINDRICAL_SURFACE('',#15308,6.05);
#1373=CYLINDRICAL_SURFACE('',#15312,6.05);
#1374=CYLINDRICAL_SURFACE('',#15316,6.05);
#1375=CYLINDRICAL_SURFACE('',#15332,62.5);
#1376=CYLINDRICAL_SURFACE('',#15351,62.5);
#1377=CYLINDRICAL_SURFACE('',#15367,2.);
#1378=CYLINDRICAL_SURFACE('',#15372,2.);
#1379=CYLINDRICAL_SURFACE('',#15378,2.);
#1380=CYLINDRICAL_SURFACE('',#15379,2.);
#1381=CYLINDRICAL_SURFACE('',#15380,14.);
#1382=CYLINDRICAL_SURFACE('',#15385,2.);
#1383=CYLINDRICAL_SURFACE('',#15390,2.);
#1384=CYLINDRICAL_SURFACE('',#15392,14.);
#1385=CYLINDRICAL_SURFACE('',#15396,2.);
#1386=CYLINDRICAL_SURFACE('',#15400,2.);
#1387=CYLINDRICAL_SURFACE('',#15406,50.8);
#1388=CYLINDRICAL_SURFACE('',#15407,2.);
#1389=CYLINDRICAL_SURFACE('',#15413,2.);
#1390=CYLINDRICAL_SURFACE('',#15420,2.);
#1391=CYLINDRICAL_SURFACE('',#15421,2.);
#1392=CYLINDRICAL_SURFACE('',#15423,2.);
#1393=CYLINDRICAL_SURFACE('',#15429,2.);
#1394=CYLINDRICAL_SURFACE('',#15431,2.);
#1395=CYLINDRICAL_SURFACE('',#15437,2.);
#1396=CYLINDRICAL_SURFACE('',#15439,2.);
#1397=CYLINDRICAL_SURFACE('',#15445,2.);
#1398=CYLINDRICAL_SURFACE('',#15450,2.);
#1399=CYLINDRICAL_SURFACE('',#15455,2.);
#1400=CYLINDRICAL_SURFACE('',#15459,28.);
#1401=CYLINDRICAL_SURFACE('',#15460,28.);
#1402=CYLINDRICAL_SURFACE('',#15465,50.);
#1403=CYLINDRICAL_SURFACE('',#15472,9.05);
#1404=CYLINDRICAL_SURFACE('',#15477,23.525);
#1405=CYLINDRICAL_SURFACE('',#15482,27.505);
#1406=CYLINDRICAL_SURFACE('',#15486,26.);
#1407=CYLINDRICAL_SURFACE('',#15490,28.);
#1408=CYLINDRICAL_SURFACE('',#15491,28.);
#1617=FACE_OUTER_BOUND('',#2504,.T.);
#1618=FACE_OUTER_BOUND('',#2505,.T.);
#1619=FACE_OUTER_BOUND('',#2506,.T.);
#1620=FACE_OUTER_BOUND('',#2508,.T.);
#1621=FACE_OUTER_BOUND('',#2509,.T.);
#1622=FACE_OUTER_BOUND('',#2511,.T.);
#1623=FACE_OUTER_BOUND('',#2512,.T.);
#1624=FACE_OUTER_BOUND('',#2513,.T.);
#1625=FACE_OUTER_BOUND('',#2515,.T.);
#1626=FACE_OUTER_BOUND('',#2516,.T.);
#1627=FACE_OUTER_BOUND('',#2517,.T.);
#1628=FACE_OUTER_BOUND('',#2519,.T.);
#1629=FACE_OUTER_BOUND('',#2520,.T.);
#1630=FACE_OUTER_BOUND('',#2521,.T.);
#1631=FACE_OUTER_BOUND('',#2522,.T.);
#1632=FACE_OUTER_BOUND('',#2523,.T.);
#1633=FACE_OUTER_BOUND('',#2529,.T.);
#1634=FACE_OUTER_BOUND('',#2530,.T.);
#1635=FACE_OUTER_BOUND('',#2531,.T.);
#1636=FACE_OUTER_BOUND('',#2532,.T.);
#1637=FACE_OUTER_BOUND('',#2533,.T.);
#1638=FACE_OUTER_BOUND('',#2534,.T.);
#1639=FACE_OUTER_BOUND('',#2535,.T.);
#1640=FACE_OUTER_BOUND('',#2536,.T.);
#1641=FACE_OUTER_BOUND('',#2537,.T.);
#1642=FACE_OUTER_BOUND('',#2538,.T.);
#1643=FACE_OUTER_BOUND('',#2539,.T.);
#1644=FACE_OUTER_BOUND('',#2540,.T.);
#1645=FACE_OUTER_BOUND('',#2541,.T.);
#1646=FACE_OUTER_BOUND('',#2542,.T.);
#1647=FACE_OUTER_BOUND('',#2543,.T.);
#1648=FACE_OUTER_BOUND('',#2544,.T.);
#1649=FACE_OUTER_BOUND('',#2545,.T.);
#1650=FACE_OUTER_BOUND('',#2546,.T.);
#1651=FACE_OUTER_BOUND('',#2547,.T.);
#1652=FACE_OUTER_BOUND('',#2548,.T.);
#1653=FACE_OUTER_BOUND('',#2549,.T.);
#1654=FACE_OUTER_BOUND('',#2550,.T.);
#1655=FACE_OUTER_BOUND('',#2551,.T.);
#1656=FACE_OUTER_BOUND('',#2552,.T.);
#1657=FACE_OUTER_BOUND('',#2553,.T.);
#1658=FACE_OUTER_BOUND('',#2554,.T.);
#1659=FACE_OUTER_BOUND('',#2555,.T.);
#1660=FACE_OUTER_BOUND('',#2559,.T.);
#1661=FACE_OUTER_BOUND('',#2560,.T.);
#1662=FACE_OUTER_BOUND('',#2561,.T.);
#1663=FACE_OUTER_BOUND('',#2562,.T.);
#1664=FACE_OUTER_BOUND('',#2563,.T.);
#1665=FACE_OUTER_BOUND('',#2564,.T.);
#1666=FACE_OUTER_BOUND('',#2565,.T.);
#1667=FACE_OUTER_BOUND('',#2566,.T.);
#1668=FACE_OUTER_BOUND('',#2567,.T.);
#1669=FACE_OUTER_BOUND('',#2568,.T.);
#1670=FACE_OUTER_BOUND('',#2569,.T.);
#1671=FACE_OUTER_BOUND('',#2570,.T.);
#1672=FACE_OUTER_BOUND('',#2571,.T.);
#1673=FACE_OUTER_BOUND('',#2572,.T.);
#1674=FACE_OUTER_BOUND('',#2573,.T.);
#1675=FACE_OUTER_BOUND('',#2574,.T.);
#1676=FACE_OUTER_BOUND('',#2575,.T.);
#1677=FACE_OUTER_BOUND('',#2576,.T.);
#1678=FACE_OUTER_BOUND('',#2577,.T.);
#1679=FACE_OUTER_BOUND('',#2578,.T.);
#1680=FACE_OUTER_BOUND('',#2579,.T.);
#1681=FACE_OUTER_BOUND('',#2580,.T.);
#1682=FACE_OUTER_BOUND('',#2581,.T.);
#1683=FACE_OUTER_BOUND('',#2582,.T.);
#1684=FACE_OUTER_BOUND('',#2583,.T.);
#1685=FACE_OUTER_BOUND('',#2584,.T.);
#1686=FACE_OUTER_BOUND('',#2585,.T.);
#1687=FACE_OUTER_BOUND('',#2586,.T.);
#1688=FACE_OUTER_BOUND('',#2587,.T.);
#1689=FACE_OUTER_BOUND('',#2588,.T.);
#1690=FACE_OUTER_BOUND('',#2589,.T.);
#1691=FACE_OUTER_BOUND('',#2590,.T.);
#1692=FACE_OUTER_BOUND('',#2591,.T.);
#1693=FACE_OUTER_BOUND('',#2592,.T.);
#1694=FACE_OUTER_BOUND('',#2593,.T.);
#1695=FACE_OUTER_BOUND('',#2594,.T.);
#1696=FACE_OUTER_BOUND('',#2595,.T.);
#1697=FACE_OUTER_BOUND('',#2596,.T.);
#1698=FACE_OUTER_BOUND('',#2597,.T.);
#1699=FACE_OUTER_BOUND('',#2598,.T.);
#1700=FACE_OUTER_BOUND('',#2599,.T.);
#1701=FACE_OUTER_BOUND('',#2600,.T.);
#1702=FACE_OUTER_BOUND('',#2601,.T.);
#1703=FACE_OUTER_BOUND('',#2602,.T.);
#1704=FACE_OUTER_BOUND('',#2603,.T.);
#1705=FACE_OUTER_BOUND('',#2604,.T.);
#1706=FACE_OUTER_BOUND('',#2605,.T.);
#1707=FACE_OUTER_BOUND('',#2606,.T.);
#1708=FACE_OUTER_BOUND('',#2607,.T.);
#1709=FACE_OUTER_BOUND('',#2608,.T.);
#1710=FACE_OUTER_BOUND('',#2609,.T.);
#1711=FACE_OUTER_BOUND('',#2610,.T.);
#1712=FACE_OUTER_BOUND('',#2611,.T.);
#1713=FACE_OUTER_BOUND('',#2614,.T.);
#1714=FACE_OUTER_BOUND('',#2615,.T.);
#1715=FACE_OUTER_BOUND('',#2616,.T.);
#1716=FACE_OUTER_BOUND('',#2617,.T.);
#1717=FACE_OUTER_BOUND('',#2618,.T.);
#1718=FACE_OUTER_BOUND('',#2619,.T.);
#1719=FACE_OUTER_BOUND('',#2620,.T.);
#1720=FACE_OUTER_BOUND('',#2621,.T.);
#1721=FACE_OUTER_BOUND('',#2622,.T.);
#1722=FACE_OUTER_BOUND('',#2623,.T.);
#1723=FACE_OUTER_BOUND('',#2624,.T.);
#1724=FACE_OUTER_BOUND('',#2625,.T.);
#1725=FACE_OUTER_BOUND('',#2626,.T.);
#1726=FACE_OUTER_BOUND('',#2627,.T.);
#1727=FACE_OUTER_BOUND('',#2628,.T.);
#1728=FACE_OUTER_BOUND('',#2630,.T.);
#1729=FACE_OUTER_BOUND('',#2631,.T.);
#1730=FACE_OUTER_BOUND('',#2633,.T.);
#1731=FACE_OUTER_BOUND('',#2634,.T.);
#1732=FACE_OUTER_BOUND('',#2636,.T.);
#1733=FACE_OUTER_BOUND('',#2638,.T.);
#1734=FACE_OUTER_BOUND('',#2639,.T.);
#1735=FACE_OUTER_BOUND('',#2640,.T.);
#1736=FACE_OUTER_BOUND('',#2641,.T.);
#2504=EDGE_LOOP('',(#9799,#9800,#9801,#9802));
#2505=EDGE_LOOP('',(#9803,#9804,#9805,#9806,#9807,#9808));
#2506=EDGE_LOOP('',(#9809));
#2507=EDGE_LOOP('',(#9810));
#2508=EDGE_LOOP('',(#9811,#9812,#9813,#9814));
#2509=EDGE_LOOP('',(#9815,#9816,#9817,#9818,#9819,#9820));
#2510=EDGE_LOOP('',(#9821));
#2511=EDGE_LOOP('',(#9822,#9823,#9824,#9825));
#2512=EDGE_LOOP('',(#9826,#9827,#9828,#9829));
#2513=EDGE_LOOP('',(#9830));
#2514=EDGE_LOOP('',(#9831));
#2515=EDGE_LOOP('',(#9832,#9833,#9834,#9835,#9836,#9837));
#2516=EDGE_LOOP('',(#9838,#9839,#9840,#9841));
#2517=EDGE_LOOP('',(#9842,#9843,#9844,#9845,#9846,#9847));
#2518=EDGE_LOOP('',(#9848));
#2519=EDGE_LOOP('',(#9849,#9850,#9851,#9852));
#2520=EDGE_LOOP('',(#9853,#9854,#9855,#9856));
#2521=EDGE_LOOP('',(#9857,#9858,#9859,#9860,#9861,#9862));
#2522=EDGE_LOOP('',(#9863,#9864,#9865,#9866));
#2523=EDGE_LOOP('',(#9867,#9868,#9869,#9870,#9871,#9872,#9873,#9874));
#2524=EDGE_LOOP('',(#9875));
#2525=EDGE_LOOP('',(#9876));
#2526=EDGE_LOOP('',(#9877));
#2527=EDGE_LOOP('',(#9878));
#2528=EDGE_LOOP('',(#9879));
#2529=EDGE_LOOP('',(#9880,#9881,#9882,#9883));
#2530=EDGE_LOOP('',(#9884,#9885,#9886,#9887));
#2531=EDGE_LOOP('',(#9888,#9889,#9890,#9891));
#2532=EDGE_LOOP('',(#9892,#9893,#9894,#9895));
#2533=EDGE_LOOP('',(#9896,#9897,#9898,#9899));
#2534=EDGE_LOOP('',(#9900,#9901,#9902,#9903));
#2535=EDGE_LOOP('',(#9904,#9905,#9906,#9907));
#2536=EDGE_LOOP('',(#9908,#9909,#9910,#9911,#9912));
#2537=EDGE_LOOP('',(#9913,#9914,#9915,#9916));
#2538=EDGE_LOOP('',(#9917,#9918,#9919,#9920,#9921,#9922,#9923,#9924,#9925,
#9926));
#2539=EDGE_LOOP('',(#9927,#9928,#9929,#9930));
#2540=EDGE_LOOP('',(#9931,#9932,#9933,#9934,#9935,#9936,#9937,#9938,#9939,
#9940,#9941,#9942,#9943));
#2541=EDGE_LOOP('',(#9944,#9945,#9946,#9947));
#2542=EDGE_LOOP('',(#9948,#9949,#9950,#9951,#9952));
#2543=EDGE_LOOP('',(#9953,#9954,#9955,#9956));
#2544=EDGE_LOOP('',(#9957,#9958,#9959,#9960,#9961,#9962,#9963,#9964,#9965,
#9966,#9967,#9968,#9969,#9970,#9971,#9972,#9973,#9974));
#2545=EDGE_LOOP('',(#9975,#9976,#9977,#9978,#9979));
#2546=EDGE_LOOP('',(#9980,#9981,#9982,#9983));
#2547=EDGE_LOOP('',(#9984,#9985,#9986,#9987,#9988,#9989,#9990,#9991,#9992,
#9993));
#2548=EDGE_LOOP('',(#9994,#9995,#9996,#9997));
#2549=EDGE_LOOP('',(#9998,#9999,#10000,#10001,#10002,#10003,#10004,#10005,
#10006,#10007,#10008,#10009,#10010));
#2550=EDGE_LOOP('',(#10011,#10012,#10013,#10014));
#2551=EDGE_LOOP('',(#10015,#10016,#10017,#10018,#10019));
#2552=EDGE_LOOP('',(#10020,#10021,#10022,#10023));
#2553=EDGE_LOOP('',(#10024,#10025,#10026,#10027,#10028,#10029,#10030,#10031,
#10032,#10033,#10034,#10035,#10036,#10037,#10038,#10039,#10040,#10041));
#2554=EDGE_LOOP('',(#10042,#10043,#10044,#10045));
#2555=EDGE_LOOP('',(#10046,#10047,#10048,#10049,#10050,#10051,#10052,#10053));
#2556=EDGE_LOOP('',(#10054));
#2557=EDGE_LOOP('',(#10055));
#2558=EDGE_LOOP('',(#10056));
#2559=EDGE_LOOP('',(#10057,#10058,#10059,#10060));
#2560=EDGE_LOOP('',(#10061,#10062,#10063,#10064));
#2561=EDGE_LOOP('',(#10065,#10066,#10067,#10068));
#2562=EDGE_LOOP('',(#10069,#10070,#10071,#10072));
#2563=EDGE_LOOP('',(#10073,#10074,#10075,#10076));
#2564=EDGE_LOOP('',(#10077,#10078,#10079,#10080));
#2565=EDGE_LOOP('',(#10081,#10082,#10083,#10084));
#2566=EDGE_LOOP('',(#10085,#10086,#10087,#10088));
#2567=EDGE_LOOP('',(#10089,#10090,#10091,#10092));
#2568=EDGE_LOOP('',(#10093,#10094,#10095,#10096));
#2569=EDGE_LOOP('',(#10097,#10098,#10099,#10100));
#2570=EDGE_LOOP('',(#10101,#10102,#10103,#10104,#10105,#10106));
#2571=EDGE_LOOP('',(#10107,#10108,#10109,#10110,#10111));
#2572=EDGE_LOOP('',(#10112,#10113,#10114,#10115));
#2573=EDGE_LOOP('',(#10116,#10117,#10118,#10119,#10120));
#2574=EDGE_LOOP('',(#10121,#10122,#10123,#10124));
#2575=EDGE_LOOP('',(#10125,#10126,#10127,#10128));
#2576=EDGE_LOOP('',(#10129,#10130,#10131,#10132));
#2577=EDGE_LOOP('',(#10133,#10134,#10135,#10136,#10137,#10138));
#2578=EDGE_LOOP('',(#10139,#10140,#10141,#10142,#10143));
#2579=EDGE_LOOP('',(#10144,#10145,#10146,#10147));
#2580=EDGE_LOOP('',(#10148,#10149,#10150,#10151,#10152));
#2581=EDGE_LOOP('',(#10153,#10154,#10155,#10156));
#2582=EDGE_LOOP('',(#10157,#10158,#10159,#10160));
#2583=EDGE_LOOP('',(#10161,#10162,#10163,#10164));
#2584=EDGE_LOOP('',(#10165,#10166,#10167,#10168,#10169));
#2585=EDGE_LOOP('',(#10170,#10171,#10172,#10173));
#2586=EDGE_LOOP('',(#10174,#10175,#10176,#10177,#10178));
#2587=EDGE_LOOP('',(#10179,#10180,#10181,#10182));
#2588=EDGE_LOOP('',(#10183,#10184,#10185,#10186));
#2589=EDGE_LOOP('',(#10187,#10188,#10189,#10190,#10191));
#2590=EDGE_LOOP('',(#10192,#10193,#10194,#10195,#10196));
#2591=EDGE_LOOP('',(#10197,#10198,#10199,#10200));
#2592=EDGE_LOOP('',(#10201,#10202,#10203,#10204,#10205));
#2593=EDGE_LOOP('',(#10206,#10207,#10208,#10209));
#2594=EDGE_LOOP('',(#10210,#10211,#10212,#10213,#10214));
#2595=EDGE_LOOP('',(#10215,#10216,#10217,#10218));
#2596=EDGE_LOOP('',(#10219,#10220,#10221,#10222,#10223));
#2597=EDGE_LOOP('',(#10224,#10225,#10226,#10227));
#2598=EDGE_LOOP('',(#10228,#10229,#10230,#10231,#10232));
#2599=EDGE_LOOP('',(#10233,#10234,#10235,#10236));
#2600=EDGE_LOOP('',(#10237,#10238,#10239,#10240));
#2601=EDGE_LOOP('',(#10241,#10242,#10243,#10244));
#2602=EDGE_LOOP('',(#10245,#10246,#10247,#10248));
#2603=EDGE_LOOP('',(#10249,#10250,#10251,#10252));
#2604=EDGE_LOOP('',(#10253,#10254,#10255,#10256));
#2605=EDGE_LOOP('',(#10257,#10258,#10259,#10260));
#2606=EDGE_LOOP('',(#10261,#10262,#10263,#10264));
#2607=EDGE_LOOP('',(#10265,#10266,#10267,#10268));
#2608=EDGE_LOOP('',(#10269,#10270,#10271,#10272,#10273,#10274));
#2609=EDGE_LOOP('',(#10275,#10276,#10277,#10278,#10279,#10280));
#2610=EDGE_LOOP('',(#10281,#10282,#10283,#10284,#10285));
#2611=EDGE_LOOP('',(#10286,#10287,#10288,#10289,#10290));
#2612=EDGE_LOOP('',(#10291,#10292,#10293,#10294));
#2613=EDGE_LOOP('',(#10295,#10296,#10297,#10298));
#2614=EDGE_LOOP('',(#10299,#10300,#10301));
#2615=EDGE_LOOP('',(#10302,#10303,#10304,#10305));
#2616=EDGE_LOOP('',(#10306,#10307,#10308));
#2617=EDGE_LOOP('',(#10309,#10310,#10311,#10312,#10313));
#2618=EDGE_LOOP('',(#10314,#10315,#10316));
#2619=EDGE_LOOP('',(#10317,#10318,#10319,#10320));
#2620=EDGE_LOOP('',(#10321,#10322,#10323));
#2621=EDGE_LOOP('',(#10324,#10325,#10326,#10327,#10328));
#2622=EDGE_LOOP('',(#10329,#10330,#10331,#10332,#10333,#10334));
#2623=EDGE_LOOP('',(#10335));
#2624=EDGE_LOOP('',(#10336));
#2625=EDGE_LOOP('',(#10337));
#2626=EDGE_LOOP('',(#10338));
#2627=EDGE_LOOP('',(#10339,#10340,#10341,#10342));
#2628=EDGE_LOOP('',(#10343));
#2629=EDGE_LOOP('',(#10344));
#2630=EDGE_LOOP('',(#10345,#10346,#10347,#10348));
#2631=EDGE_LOOP('',(#10349));
#2632=EDGE_LOOP('',(#10350));
#2633=EDGE_LOOP('',(#10351,#10352,#10353,#10354));
#2634=EDGE_LOOP('',(#10355));
#2635=EDGE_LOOP('',(#10356));
#2636=EDGE_LOOP('',(#10357));
#2637=EDGE_LOOP('',(#10358));
#2638=EDGE_LOOP('',(#10359,#10360,#10361,#10362));
#2639=EDGE_LOOP('',(#10363,#10364,#10365,#10366));
#2640=EDGE_LOOP('',(#10367,#10368));
#2641=EDGE_LOOP('',(#10369,#10370));
#3532=LINE('',#20896,#4601);
#3533=LINE('',#20900,#4602);
#3534=LINE('',#20922,#4603);
#3535=LINE('',#20927,#4604);
#3536=LINE('',#20931,#4605);
#3537=LINE('',#20935,#4606);
#3538=LINE('',#20940,#4607);
#3539=LINE('',#20945,#4608);
#3540=LINE('',#20952,#4609);
#3541=LINE('',#20971,#4610);
#3542=LINE('',#20976,#4611);
#3543=LINE('',#20980,#4612);
#3544=LINE('',#20984,#4613);
#3545=LINE('',#20989,#4614);
#3546=LINE('',#20992,#4615);
#3547=LINE('',#20996,#4616);
#3548=LINE('',#21018,#4617);
#3549=LINE('',#21023,#4618);
#3550=LINE('',#21027,#4619);
#3551=LINE('',#21031,#4620);
#3552=LINE('',#21035,#4621);
#3553=LINE('',#21047,#4622);
#3554=LINE('',#21051,#4623);
#3555=LINE('',#21055,#4624);
#3556=LINE('',#21059,#4625);
#3557=LINE('',#21063,#4626);
#3558=LINE('',#21067,#4627);
#3559=LINE('',#21071,#4628);
#3560=LINE('',#21095,#4629);
#3561=LINE('',#21098,#4630);
#3562=LINE('',#21101,#4631);
#3563=LINE('',#21103,#4632);
#3564=LINE('',#21105,#4633);
#3565=LINE('',#21107,#4634);
#3566=LINE('',#21109,#4635);
#3567=LINE('',#21111,#4636);
#3568=LINE('',#21129,#4637);
#3569=LINE('',#21132,#4638);
#3570=LINE('',#21135,#4639);
#3571=LINE('',#21148,#4640);
#3572=LINE('',#21161,#4641);
#3573=LINE('',#21163,#4642);
#3574=LINE('',#21164,#4643);
#3575=LINE('',#21166,#4644);
#3576=LINE('',#21168,#4645);
#3577=LINE('',#21169,#4646);
#3578=LINE('',#21184,#4647);
#3579=LINE('',#21207,#4648);
#3580=LINE('',#21210,#4649);
#3581=LINE('',#21222,#4650);
#3582=LINE('',#21226,#4651);
#3583=LINE('',#21296,#4652);
#3584=LINE('',#21299,#4653);
#3585=LINE('',#21302,#4654);
#3586=LINE('',#21304,#4655);
#3587=LINE('',#21306,#4656);
#3588=LINE('',#21308,#4657);
#3589=LINE('',#21309,#4658);
#3590=LINE('',#21324,#4659);
#3591=LINE('',#21327,#4660);
#3592=LINE('',#21330,#4661);
#3593=LINE('',#21343,#4662);
#3594=LINE('',#21356,#4663);
#3595=LINE('',#21358,#4664);
#3596=LINE('',#21360,#4665);
#3597=LINE('',#21362,#4666);
#3598=LINE('',#21363,#4667);
#3599=LINE('',#21364,#4668);
#3600=LINE('',#21379,#4669);
#3601=LINE('',#21399,#4670);
#3602=LINE('',#21411,#4671);
#3603=LINE('',#21415,#4672);
#3604=LINE('',#21466,#4673);
#3605=LINE('',#21472,#4674);
#3606=LINE('',#21476,#4675);
#3607=LINE('',#21480,#4676);
#3608=LINE('',#21483,#4677);
#3609=LINE('',#21489,#4678);
#3610=LINE('',#21522,#4679);
#3611=LINE('',#21542,#4680);
#3612=LINE('',#21565,#4681);
#3613=LINE('',#21567,#4682);
#3614=LINE('',#21570,#4683);
#3615=LINE('',#21573,#4684);
#3616=LINE('',#21575,#4685);
#3617=LINE('',#21581,#4686);
#3618=LINE('',#21587,#4687);
#3619=LINE('',#21589,#4688);
#3620=LINE('',#21591,#4689);
#3621=LINE('',#21597,#4690);
#3622=LINE('',#21609,#4691);
#3623=LINE('',#21612,#4692);
#3624=LINE('',#21620,#4693);
#3625=LINE('',#21630,#4694);
#3626=LINE('',#21632,#4695);
#3627=LINE('',#21636,#4696);
#3628=LINE('',#21644,#4697);
#3629=LINE('',#21648,#4698);
#3630=LINE('',#21656,#4699);
#3631=LINE('',#21689,#4700);
#3632=LINE('',#22595,#4701);
#3633=LINE('',#22604,#4702);
#3634=LINE('',#22611,#4703);
#3635=LINE('',#22618,#4704);
#4601=VECTOR('',#16783,14.75);
#4602=VECTOR('',#16788,15.);
#4603=VECTOR('',#16801,7.4);
#4604=VECTOR('',#16806,10.);
#4605=VECTOR('',#16809,10.);
#4606=VECTOR('',#16812,10.);
#4607=VECTOR('',#16819,7.15);
#4608=VECTOR('',#16824,14.75);
#4609=VECTOR('',#16833,15.);
#4610=VECTOR('',#16842,7.4);
#4611=VECTOR('',#16847,10.);
#4612=VECTOR('',#16850,10.);
#4613=VECTOR('',#16853,10.);
#4614=VECTOR('',#16860,7.15);
#4615=VECTOR('',#16863,9.3);
#4616=VECTOR('',#16868,9.05);
#4617=VECTOR('',#16875,6.3);
#4618=VECTOR('',#16880,10.);
#4619=VECTOR('',#16883,10.);
#4620=VECTOR('',#16886,10.);
#4621=VECTOR('',#16889,10.);
#4622=VECTOR('',#16902,6.05);
#4623=VECTOR('',#16907,6.3);
#4624=VECTOR('',#16912,6.05);
#4625=VECTOR('',#16917,6.3);
#4626=VECTOR('',#16922,6.05);
#4627=VECTOR('',#16927,6.3);
#4628=VECTOR('',#16932,6.05);
#4629=VECTOR('',#16941,10.);
#4630=VECTOR('',#16944,10.);
#4631=VECTOR('',#16947,10.);
#4632=VECTOR('',#16948,10.);
#4633=VECTOR('',#16949,10.);
#4634=VECTOR('',#16950,10.);
#4635=VECTOR('',#16951,10.);
#4636=VECTOR('',#16952,10.);
#4637=VECTOR('',#16955,10.);
#4638=VECTOR('',#16958,10.);
#4639=VECTOR('',#16961,10.);
#4640=VECTOR('',#16962,10.);
#4641=VECTOR('',#16963,10.);
#4642=VECTOR('',#16964,10.);
#4643=VECTOR('',#16965,10.);
#4644=VECTOR('',#16966,10.);
#4645=VECTOR('',#16967,10.);
#4646=VECTOR('',#16968,10.);
#4647=VECTOR('',#16973,10.);
#4648=VECTOR('',#16980,10.);
#4649=VECTOR('',#16983,10.);
#4650=VECTOR('',#16986,10.);
#4651=VECTOR('',#16989,10.);
#4652=VECTOR('',#17002,10.);
#4653=VECTOR('',#17005,10.);
#4654=VECTOR('',#17008,10.);
#4655=VECTOR('',#17009,10.);
#4656=VECTOR('',#17010,10.);
#4657=VECTOR('',#17011,10.);
#4658=VECTOR('',#17012,10.);
#4659=VECTOR('',#17015,10.);
#4660=VECTOR('',#17018,10.);
#4661=VECTOR('',#17021,10.);
#4662=VECTOR('',#17022,10.);
#4663=VECTOR('',#17023,10.);
#4664=VECTOR('',#17024,10.);
#4665=VECTOR('',#17025,10.);
#4666=VECTOR('',#17026,10.);
#4667=VECTOR('',#17027,10.);
#4668=VECTOR('',#17028,10.);
#4669=VECTOR('',#17033,10.);
#4670=VECTOR('',#17042,10.);
#4671=VECTOR('',#17045,10.);
#4672=VECTOR('',#17048,10.);
#4673=VECTOR('',#17059,7.4);
#4674=VECTOR('',#17064,10.);
#4675=VECTOR('',#17067,10.);
#4676=VECTOR('',#17070,10.);
#4677=VECTOR('',#17073,10.);
#4678=VECTOR('',#17080,7.4);
#4679=VECTOR('',#17087,10.);
#4680=VECTOR('',#17096,10.);
#4681=VECTOR('',#17109,10.);
#4682=VECTOR('',#17112,10.);
#4683=VECTOR('',#17115,10.);
#4684=VECTOR('',#17118,10.);
#4685=VECTOR('',#17121,10.);
#4686=VECTOR('',#17130,10.);
#4687=VECTOR('',#17139,10.);
#4688=VECTOR('',#17142,10.);
#4689=VECTOR('',#17145,10.);
#4690=VECTOR('',#17156,10.);
#4691=VECTOR('',#17175,50.8);
#4692=VECTOR('',#17178,10.);
#4693=VECTOR('',#17191,10.);
#4694=VECTOR('',#17206,10.);
#4695=VECTOR('',#17209,10.);
#4696=VECTOR('',#17214,10.);
#4697=VECTOR('',#17227,10.);
#4698=VECTOR('',#17232,10.);
#4699=VECTOR('',#17245,10.);
#4700=VECTOR('',#17304,50.);
#4701=VECTOR('',#17317,9.05);
#4702=VECTOR('',#17330,23.525);
#4703=VECTOR('',#17339,27.505);
#4704=VECTOR('',#17348,26.);
#5670=CIRCLE('',#15255,14.5);
#5671=CIRCLE('',#15256,15.);
#5672=CIRCLE('',#15258,15.);
#5673=CIRCLE('',#15259,15.);
#5674=CIRCLE('',#15261,9.05);
#5675=CIRCLE('',#15263,7.65);
#5676=CIRCLE('',#15264,7.15);
#5677=CIRCLE('',#15266,62.);
#5678=CIRCLE('',#15267,62.);
#5679=CIRCLE('',#15268,12.);
#5680=CIRCLE('',#15270,7.15);
#5681=CIRCLE('',#15272,14.5);
#5682=CIRCLE('',#15273,15.);
#5683=CIRCLE('',#15275,9.55);
#5684=CIRCLE('',#15277,15.);
#5685=CIRCLE('',#15278,15.);
#5686=CIRCLE('',#15280,7.65);
#5687=CIRCLE('',#15281,7.15);
#5688=CIRCLE('',#15283,12.);
#5689=CIRCLE('',#15284,62.);
#5690=CIRCLE('',#15285,62.);
#5691=CIRCLE('',#15287,7.15);
#5692=CIRCLE('',#15289,9.05);
#5693=CIRCLE('',#15291,9.05);
#5694=CIRCLE('',#15293,6.55);
#5695=CIRCLE('',#15294,6.05);
#5696=CIRCLE('',#15296,26.);
#5697=CIRCLE('',#15297,26.);
#5698=CIRCLE('',#15298,26.);
#5699=CIRCLE('',#15299,26.);
#5700=CIRCLE('',#15300,6.55);
#5701=CIRCLE('',#15301,6.55);
#5702=CIRCLE('',#15302,52.);
#5703=CIRCLE('',#15303,6.55);
#5704=CIRCLE('',#15305,6.05);
#5705=CIRCLE('',#15307,6.05);
#5706=CIRCLE('',#15309,6.05);
#5707=CIRCLE('',#15311,6.05);
#5708=CIRCLE('',#15313,6.05);
#5709=CIRCLE('',#15315,6.05);
#5710=CIRCLE('',#15317,6.05);
#5711=CIRCLE('',#15319,62.5);
#5712=CIRCLE('',#15329,62.5);
#5713=CIRCLE('',#15333,62.5);
#5714=CIRCLE('',#15334,62.5);
#5715=CIRCLE('',#15335,62.5);
#5716=CIRCLE('',#15336,62.5);
#5717=CIRCLE('',#15338,62.5);
#5718=CIRCLE('',#15348,62.5);
#5719=CIRCLE('',#15352,62.5);
#5720=CIRCLE('',#15353,62.5);
#5721=CIRCLE('',#15354,62.5);
#5722=CIRCLE('',#15355,62.5);
#5723=CIRCLE('',#15357,7.65);
#5724=CIRCLE('',#15359,60.5);
#5725=CIRCLE('',#15360,12.);
#5726=CIRCLE('',#15361,60.5);
#5727=CIRCLE('',#15362,12.);
#5728=CIRCLE('',#15363,7.65);
#5729=CIRCLE('',#15364,50.8);
#5730=CIRCLE('',#15368,2.);
#5731=CIRCLE('',#15370,2.);
#5732=CIRCLE('',#15371,14.);
#5733=CIRCLE('',#15375,2.);
#5734=CIRCLE('',#15376,2.);
#5735=CIRCLE('',#15377,14.);
#5736=CIRCLE('',#15381,14.);
#5737=CIRCLE('',#15384,60.5);
#5738=CIRCLE('',#15386,2.);
#5739=CIRCLE('',#15388,2.);
#5740=CIRCLE('',#15389,14.);
#5741=CIRCLE('',#15395,60.5);
#5742=CIRCLE('',#15397,2.);
#5743=CIRCLE('',#15399,2.);
#5744=CIRCLE('',#15403,50.8);
#5745=CIRCLE('',#15404,2.);
#5746=CIRCLE('',#15405,50.3);
#5747=CIRCLE('',#15408,2.);
#5748=CIRCLE('',#15410,2.);
#5749=CIRCLE('',#15411,28.);
#5750=CIRCLE('',#15412,26.);
#5751=CIRCLE('',#15416,2.);
#5752=CIRCLE('',#15417,26.);
#5753=CIRCLE('',#15418,2.);
#5754=CIRCLE('',#15419,28.);
#5755=CIRCLE('',#15424,2.);
#5756=CIRCLE('',#15426,2.);
#5757=CIRCLE('',#15427,28.);
#5758=CIRCLE('',#15428,26.);
#5759=CIRCLE('',#15432,2.);
#5760=CIRCLE('',#15434,2.);
#5761=CIRCLE('',#15435,28.);
#5762=CIRCLE('',#15436,26.);
#5763=CIRCLE('',#15440,1.99999999999999);
#5764=CIRCLE('',#15441,2.);
#5765=CIRCLE('',#15443,2.);
#5766=CIRCLE('',#15444,28.);
#5767=CIRCLE('',#15446,2.);
#5768=CIRCLE('',#15448,2.);
#5769=CIRCLE('',#15449,28.);
#5770=CIRCLE('',#15451,2.);
#5771=CIRCLE('',#15453,2.);
#5772=CIRCLE('',#15454,28.);
#5773=CIRCLE('',#15456,2.);
#5774=CIRCLE('',#15458,28.);
#5775=CIRCLE('',#15462,2.);
#5776=CIRCLE('',#15463,50.);
#5777=CIRCLE('',#15464,50.);
#5778=CIRCLE('',#15466,50.);
#5779=CIRCLE('',#15467,2.00000000000001);
#5780=CIRCLE('',#15468,2.);
#5781=CIRCLE('',#15469,1.99999999999999);
#5782=CIRCLE('',#15470,1.99999999999999);
#5783=CIRCLE('',#15471,9.05);
#5784=CIRCLE('',#15478,23.525);
#5785=CIRCLE('',#15479,23.525);
#5786=CIRCLE('',#15481,27.505);
#5787=CIRCLE('',#15483,27.505);
#5788=CIRCLE('',#15485,26.);
#5789=CIRCLE('',#15487,26.);
#6271=VERTEX_POINT('',#20893);
#6272=VERTEX_POINT('',#20895);
#6273=VERTEX_POINT('',#20899);
#6274=VERTEX_POINT('',#20901);
#6275=VERTEX_POINT('',#20903);
#6276=VERTEX_POINT('',#20916);
#6277=VERTEX_POINT('',#20919);
#6278=VERTEX_POINT('',#20921);
#6279=VERTEX_POINT('',#20925);
#6280=VERTEX_POINT('',#20926);
#6281=VERTEX_POINT('',#20928);
#6282=VERTEX_POINT('',#20930);
#6283=VERTEX_POINT('',#20932);
#6284=VERTEX_POINT('',#20934);
#6285=VERTEX_POINT('',#20938);
#6286=VERTEX_POINT('',#20942);
#6287=VERTEX_POINT('',#20944);
#6288=VERTEX_POINT('',#20948);
#6289=VERTEX_POINT('',#20951);
#6290=VERTEX_POINT('',#20953);
#6291=VERTEX_POINT('',#20955);
#6292=VERTEX_POINT('',#20968);
#6293=VERTEX_POINT('',#20970);
#6294=VERTEX_POINT('',#20974);
#6295=VERTEX_POINT('',#20975);
#6296=VERTEX_POINT('',#20977);
#6297=VERTEX_POINT('',#20979);
#6298=VERTEX_POINT('',#20981);
#6299=VERTEX_POINT('',#20983);
#6300=VERTEX_POINT('',#20987);
#6301=VERTEX_POINT('',#20991);
#6302=VERTEX_POINT('',#20995);
#6303=VERTEX_POINT('',#20997);
#6304=VERTEX_POINT('',#21003);
#6305=VERTEX_POINT('',#21015);
#6306=VERTEX_POINT('',#21017);
#6307=VERTEX_POINT('',#21021);
#6308=VERTEX_POINT('',#21022);
#6309=VERTEX_POINT('',#21024);
#6310=VERTEX_POINT('',#21026);
#6311=VERTEX_POINT('',#21028);
#6312=VERTEX_POINT('',#21030);
#6313=VERTEX_POINT('',#21032);
#6314=VERTEX_POINT('',#21034);
#6315=VERTEX_POINT('',#21037);
#6316=VERTEX_POINT('',#21039);
#6317=VERTEX_POINT('',#21041);
#6318=VERTEX_POINT('',#21043);
#6319=VERTEX_POINT('',#21046);
#6320=VERTEX_POINT('',#21050);
#6321=VERTEX_POINT('',#21054);
#6322=VERTEX_POINT('',#21058);
#6323=VERTEX_POINT('',#21062);
#6324=VERTEX_POINT('',#21066);
#6325=VERTEX_POINT('',#21070);
#6326=VERTEX_POINT('',#21074);
#6327=VERTEX_POINT('',#21083);
#6328=VERTEX_POINT('',#21085);
#6329=VERTEX_POINT('',#21094);
#6330=VERTEX_POINT('',#21096);
#6331=VERTEX_POINT('',#21100);
#6332=VERTEX_POINT('',#21102);
#6333=VERTEX_POINT('',#21104);
#6334=VERTEX_POINT('',#21106);
#6335=VERTEX_POINT('',#21108);
#6336=VERTEX_POINT('',#21110);
#6337=VERTEX_POINT('',#21116);
#6338=VERTEX_POINT('',#21117);
#6339=VERTEX_POINT('',#21128);
#6340=VERTEX_POINT('',#21130);
#6341=VERTEX_POINT('',#21134);
#6342=VERTEX_POINT('',#21136);
#6343=VERTEX_POINT('',#21147);
#6344=VERTEX_POINT('',#21149);
#6345=VERTEX_POINT('',#21160);
#6346=VERTEX_POINT('',#21162);
#6347=VERTEX_POINT('',#21165);
#6348=VERTEX_POINT('',#21167);
#6349=VERTEX_POINT('',#21171);
#6350=VERTEX_POINT('',#21173);
#6351=VERTEX_POINT('',#21186);
#6352=VERTEX_POINT('',#21187);
#6353=VERTEX_POINT('',#21197);
#6354=VERTEX_POINT('',#21206);
#6355=VERTEX_POINT('',#21208);
#6356=VERTEX_POINT('',#21212);
#6357=VERTEX_POINT('',#21221);
#6358=VERTEX_POINT('',#21223);
#6359=VERTEX_POINT('',#21225);
#6360=VERTEX_POINT('',#21235);
#6361=VERTEX_POINT('',#21244);
#6362=VERTEX_POINT('',#21255);
#6363=VERTEX_POINT('',#21264);
#6364=VERTEX_POINT('',#21275);
#6365=VERTEX_POINT('',#21284);
#6366=VERTEX_POINT('',#21286);
#6367=VERTEX_POINT('',#21295);
#6368=VERTEX_POINT('',#21297);
#6369=VERTEX_POINT('',#21301);
#6370=VERTEX_POINT('',#21303);
#6371=VERTEX_POINT('',#21305);
#6372=VERTEX_POINT('',#21307);
#6373=VERTEX_POINT('',#21311);
#6374=VERTEX_POINT('',#21312);
#6375=VERTEX_POINT('',#21323);
#6376=VERTEX_POINT('',#21325);
#6377=VERTEX_POINT('',#21329);
#6378=VERTEX_POINT('',#21331);
#6379=VERTEX_POINT('',#21342);
#6380=VERTEX_POINT('',#21344);
#6381=VERTEX_POINT('',#21355);
#6382=VERTEX_POINT('',#21357);
#6383=VERTEX_POINT('',#21359);
#6384=VERTEX_POINT('',#21361);
#6385=VERTEX_POINT('',#21366);
#6386=VERTEX_POINT('',#21368);
#6387=VERTEX_POINT('',#21381);
#6388=VERTEX_POINT('',#21382);
#6389=VERTEX_POINT('',#21397);
#6390=VERTEX_POINT('',#21401);
#6391=VERTEX_POINT('',#21410);
#6392=VERTEX_POINT('',#21412);
#6393=VERTEX_POINT('',#21414);
#6394=VERTEX_POINT('',#21424);
#6395=VERTEX_POINT('',#21433);
#6396=VERTEX_POINT('',#21444);
#6397=VERTEX_POINT('',#21453);
#6398=VERTEX_POINT('',#21464);
#6399=VERTEX_POINT('',#21468);
#6400=VERTEX_POINT('',#21469);
#6401=VERTEX_POINT('',#21471);
#6402=VERTEX_POINT('',#21473);
#6403=VERTEX_POINT('',#21475);
#6404=VERTEX_POINT('',#21477);
#6405=VERTEX_POINT('',#21479);
#6406=VERTEX_POINT('',#21481);
#6407=VERTEX_POINT('',#21484);
#6408=VERTEX_POINT('',#21486);
#6409=VERTEX_POINT('',#21520);
#6410=VERTEX_POINT('',#21524);
#6411=VERTEX_POINT('',#21559);
#6412=VERTEX_POINT('',#21561);
#6413=VERTEX_POINT('',#21569);
#6414=VERTEX_POINT('',#21571);
#6415=VERTEX_POINT('',#21579);
#6416=VERTEX_POINT('',#21583);
#6417=VERTEX_POINT('',#21603);
#6418=VERTEX_POINT('',#21605);
#6419=VERTEX_POINT('',#21611);
#6420=VERTEX_POINT('',#21615);
#6421=VERTEX_POINT('',#21623);
#6422=VERTEX_POINT('',#21625);
#6423=VERTEX_POINT('',#21635);
#6424=VERTEX_POINT('',#21639);
#6425=VERTEX_POINT('',#21647);
#6426=VERTEX_POINT('',#21651);
#6427=VERTEX_POINT('',#21681);
#6428=VERTEX_POINT('',#21683);
#6429=VERTEX_POINT('',#21687);
#6430=VERTEX_POINT('',#21690);
#6431=VERTEX_POINT('',#21691);
#6432=VERTEX_POINT('',#21717);
#6433=VERTEX_POINT('',#21728);
#6434=VERTEX_POINT('',#21890);
#6435=VERTEX_POINT('',#21891);
#6436=VERTEX_POINT('',#21898);
#6437=VERTEX_POINT('',#21909);
#6438=VERTEX_POINT('',#22398);
#6439=VERTEX_POINT('',#22482);
#6440=VERTEX_POINT('',#22579);
#6441=VERTEX_POINT('',#22601);
#6442=VERTEX_POINT('',#22603);
#6443=VERTEX_POINT('',#22607);
#6444=VERTEX_POINT('',#22610);
#6445=VERTEX_POINT('',#22614);
#6446=VERTEX_POINT('',#22617);
#7648=EDGE_CURVE('',#6271,#6271,#5670,.T.);
#7649=EDGE_CURVE('',#6271,#6272,#3532,.T.);
#7650=EDGE_CURVE('',#6272,#6272,#5671,.T.);
#7651=EDGE_CURVE('',#6272,#6273,#3533,.T.);
#7652=EDGE_CURVE('',#6274,#6273,#5672,.T.);
#7653=EDGE_CURVE('',#6275,#6274,#1009,.T.);
#7654=EDGE_CURVE('',#6273,#6275,#5673,.T.);
#7655=EDGE_CURVE('',#6276,#6276,#5674,.T.);
#7656=EDGE_CURVE('',#6277,#6277,#5675,.T.);
#7657=EDGE_CURVE('',#6277,#6278,#3534,.T.);
#7658=EDGE_CURVE('',#6278,#6278,#5676,.T.);
#7659=EDGE_CURVE('',#6279,#6280,#3535,.T.);
#7660=EDGE_CURVE('',#6281,#6279,#5677,.T.);
#7661=EDGE_CURVE('',#6281,#6282,#3536,.T.);
#7662=EDGE_CURVE('',#6283,#6282,#5678,.T.);
#7663=EDGE_CURVE('',#6284,#6283,#3537,.T.);
#7664=EDGE_CURVE('',#6280,#6284,#5679,.T.);
#7665=EDGE_CURVE('',#6285,#6285,#5680,.T.);
#7666=EDGE_CURVE('',#6285,#6278,#3538,.T.);
#7667=EDGE_CURVE('',#6286,#6286,#5681,.T.);
#7668=EDGE_CURVE('',#6286,#6287,#3539,.T.);
#7669=EDGE_CURVE('',#6287,#6287,#5682,.T.);
#7670=EDGE_CURVE('',#6288,#6288,#5683,.T.);
#7671=EDGE_CURVE('',#6287,#6289,#3540,.T.);
#7672=EDGE_CURVE('',#6290,#6289,#5684,.T.);
#7673=EDGE_CURVE('',#6291,#6290,#1010,.T.);
#7674=EDGE_CURVE('',#6289,#6291,#5685,.T.);
#7675=EDGE_CURVE('',#6292,#6292,#5686,.T.);
#7676=EDGE_CURVE('',#6292,#6293,#3541,.T.);
#7677=EDGE_CURVE('',#6293,#6293,#5687,.T.);
#7678=EDGE_CURVE('',#6294,#6295,#3542,.T.);
#7679=EDGE_CURVE('',#6296,#6294,#5688,.T.);
#7680=EDGE_CURVE('',#6297,#6296,#3543,.T.);
#7681=EDGE_CURVE('',#6298,#6297,#5689,.T.);
#7682=EDGE_CURVE('',#6298,#6299,#3544,.T.);
#7683=EDGE_CURVE('',#6295,#6299,#5690,.T.);
#7684=EDGE_CURVE('',#6300,#6300,#5691,.T.);
#7685=EDGE_CURVE('',#6300,#6293,#3545,.T.);
#7686=EDGE_CURVE('',#6288,#6301,#3546,.T.);
#7687=EDGE_CURVE('',#6301,#6301,#5692,.T.);
#7688=EDGE_CURVE('',#6301,#6302,#3547,.T.);
#7689=EDGE_CURVE('',#6303,#6302,#1011,.T.);
#7690=EDGE_CURVE('',#6303,#6304,#5693,.T.);
#7691=EDGE_CURVE('',#6302,#6304,#1012,.T.);
#7692=EDGE_CURVE('',#6305,#6305,#5694,.T.);
#7693=EDGE_CURVE('',#6305,#6306,#3548,.T.);
#7694=EDGE_CURVE('',#6306,#6306,#5695,.T.);
#7695=EDGE_CURVE('',#6307,#6308,#3549,.T.);
#7696=EDGE_CURVE('',#6309,#6307,#5696,.T.);
#7697=EDGE_CURVE('',#6310,#6309,#3550,.T.);
#7698=EDGE_CURVE('',#6311,#6310,#5697,.T.);
#7699=EDGE_CURVE('',#6312,#6311,#3551,.T.);
#7700=EDGE_CURVE('',#6313,#6312,#5698,.T.);
#7701=EDGE_CURVE('',#6314,#6313,#3552,.T.);
#7702=EDGE_CURVE('',#6308,#6314,#5699,.T.);
#7703=EDGE_CURVE('',#6315,#6315,#5700,.T.);
#7704=EDGE_CURVE('',#6316,#6316,#5701,.T.);
#7705=EDGE_CURVE('',#6317,#6317,#5702,.T.);
#7706=EDGE_CURVE('',#6318,#6318,#5703,.T.);
#7707=EDGE_CURVE('',#6306,#6319,#3553,.T.);
#7708=EDGE_CURVE('',#6319,#6319,#5704,.T.);
#7709=EDGE_CURVE('',#6315,#6320,#3554,.T.);
#7710=EDGE_CURVE('',#6320,#6320,#5705,.T.);
#7711=EDGE_CURVE('',#6320,#6321,#3555,.T.);
#7712=EDGE_CURVE('',#6321,#6321,#5706,.T.);
#7713=EDGE_CURVE('',#6318,#6322,#3556,.T.);
#7714=EDGE_CURVE('',#6322,#6322,#5707,.T.);
#7715=EDGE_CURVE('',#6322,#6323,#3557,.T.);
#7716=EDGE_CURVE('',#6323,#6323,#5708,.T.);
#7717=EDGE_CURVE('',#6316,#6324,#3558,.T.);
#7718=EDGE_CURVE('',#6324,#6324,#5709,.T.);
#7719=EDGE_CURVE('',#6324,#6325,#3559,.T.);
#7720=EDGE_CURVE('',#6325,#6325,#5710,.T.);
#7721=EDGE_CURVE('',#6279,#6326,#1013,.F.);
#7722=EDGE_CURVE('',#6326,#6327,#5711,.T.);
#7723=EDGE_CURVE('',#6327,#6328,#1014,.T.);
#7724=EDGE_CURVE('',#6328,#6281,#332,.T.);
#7725=EDGE_CURVE('',#6327,#6329,#3560,.T.);
#7726=EDGE_CURVE('',#6329,#6330,#293,.F.);
#7727=EDGE_CURVE('',#6330,#6328,#3561,.T.);
#7728=EDGE_CURVE('',#6331,#6330,#3562,.T.);
#7729=EDGE_CURVE('',#6331,#6332,#3563,.T.);
#7730=EDGE_CURVE('',#6333,#6332,#3564,.T.);
#7731=EDGE_CURVE('',#6334,#6333,#3565,.T.);
#7732=EDGE_CURVE('',#6335,#6334,#3566,.T.);
#7733=EDGE_CURVE('',#6336,#6335,#3567,.T.);
#7734=EDGE_CURVE('',#6282,#6336,#333,.T.);
#7735=EDGE_CURVE('',#6337,#6338,#1015,.F.);
#7736=EDGE_CURVE('',#6338,#6339,#3568,.T.);
#7737=EDGE_CURVE('',#6339,#6340,#294,.F.);
#7738=EDGE_CURVE('',#6340,#6337,#3569,.T.);
#7739=EDGE_CURVE('',#6339,#6341,#3570,.T.);
#7740=EDGE_CURVE('',#6342,#6338,#1016,.F.);
#7741=EDGE_CURVE('',#6343,#6342,#3571,.T.);
#7742=EDGE_CURVE('',#6344,#6343,#1017,.F.);
#7743=EDGE_CURVE('',#6345,#6344,#3572,.T.);
#7744=EDGE_CURVE('',#6346,#6345,#3573,.T.);
#7745=EDGE_CURVE('',#6346,#6274,#3574,.T.);
#7746=EDGE_CURVE('',#6275,#6347,#3575,.T.);
#7747=EDGE_CURVE('',#6348,#6347,#3576,.T.);
#7748=EDGE_CURVE('',#6341,#6348,#3577,.T.);
#7749=EDGE_CURVE('',#6349,#6345,#295,.F.);
#7750=EDGE_CURVE('',#6344,#6350,#1018,.F.);
#7751=EDGE_CURVE('',#6350,#6349,#3578,.T.);
#7752=EDGE_CURVE('',#6351,#6352,#5712,.T.);
#7753=EDGE_CURVE('',#6352,#6295,#1019,.F.);
#7754=EDGE_CURVE('',#6299,#6353,#334,.T.);
#7755=EDGE_CURVE('',#6353,#6351,#1020,.T.);
#7756=EDGE_CURVE('',#6353,#6354,#3579,.T.);
#7757=EDGE_CURVE('',#6354,#6355,#296,.F.);
#7758=EDGE_CURVE('',#6355,#6351,#3580,.T.);
#7759=EDGE_CURVE('',#6356,#6326,#1021,.F.);
#7760=EDGE_CURVE('',#6357,#6356,#3581,.T.);
#7761=EDGE_CURVE('',#6358,#6357,#5713,.T.);
#7762=EDGE_CURVE('',#6358,#6359,#3582,.T.);
#7763=EDGE_CURVE('',#6352,#6359,#1022,.F.);
#7764=EDGE_CURVE('',#6355,#6360,#1023,.T.);
#7765=EDGE_CURVE('',#6361,#6360,#5714,.T.);
#7766=EDGE_CURVE('',#6349,#6361,#1024,.F.);
#7767=EDGE_CURVE('',#6337,#6350,#5715,.T.);
#7768=EDGE_CURVE('',#6340,#6362,#1025,.T.);
#7769=EDGE_CURVE('',#6363,#6362,#5716,.T.);
#7770=EDGE_CURVE('',#6329,#6363,#1026,.F.);
#7771=EDGE_CURVE('',#6297,#6364,#1027,.F.);
#7772=EDGE_CURVE('',#6364,#6365,#5717,.T.);
#7773=EDGE_CURVE('',#6365,#6366,#1028,.T.);
#7774=EDGE_CURVE('',#6366,#6298,#335,.T.);
#7775=EDGE_CURVE('',#6365,#6367,#3583,.T.);
#7776=EDGE_CURVE('',#6367,#6368,#297,.F.);
#7777=EDGE_CURVE('',#6368,#6366,#3584,.T.);
#7778=EDGE_CURVE('',#6369,#6368,#3585,.T.);
#7779=EDGE_CURVE('',#6369,#6370,#3586,.T.);
#7780=EDGE_CURVE('',#6371,#6370,#3587,.T.);
#7781=EDGE_CURVE('',#6372,#6371,#3588,.T.);
#7782=EDGE_CURVE('',#6354,#6372,#3589,.T.);
#7783=EDGE_CURVE('',#6373,#6374,#1029,.F.);
#7784=EDGE_CURVE('',#6374,#6375,#3590,.T.);
#7785=EDGE_CURVE('',#6375,#6376,#298,.F.);
#7786=EDGE_CURVE('',#6376,#6373,#3591,.T.);
#7787=EDGE_CURVE('',#6375,#6377,#3592,.T.);
#7788=EDGE_CURVE('',#6378,#6374,#1030,.F.);
#7789=EDGE_CURVE('',#6379,#6378,#3593,.T.);
#7790=EDGE_CURVE('',#6380,#6379,#1031,.F.);
#7791=EDGE_CURVE('',#6381,#6380,#3594,.T.);
#7792=EDGE_CURVE('',#6382,#6381,#3595,.T.);
#7793=EDGE_CURVE('',#6382,#6383,#3596,.T.);
#7794=EDGE_CURVE('',#6384,#6383,#3597,.T.);
#7795=EDGE_CURVE('',#6290,#6384,#3598,.T.);
#7796=EDGE_CURVE('',#6377,#6291,#3599,.T.);
#7797=EDGE_CURVE('',#6385,#6381,#299,.F.);
#7798=EDGE_CURVE('',#6380,#6386,#1032,.F.);
#7799=EDGE_CURVE('',#6386,#6385,#3600,.T.);
#7800=EDGE_CURVE('',#6387,#6388,#5718,.T.);
#7801=EDGE_CURVE('',#6388,#6283,#1033,.F.);
#7802=EDGE_CURVE('',#6336,#6387,#1034,.T.);
#7803=EDGE_CURVE('',#6335,#6389,#300,.F.);
#7804=EDGE_CURVE('',#6389,#6387,#3601,.T.);
#7805=EDGE_CURVE('',#6390,#6364,#1035,.F.);
#7806=EDGE_CURVE('',#6391,#6390,#3602,.T.);
#7807=EDGE_CURVE('',#6392,#6391,#5719,.T.);
#7808=EDGE_CURVE('',#6392,#6393,#3603,.T.);
#7809=EDGE_CURVE('',#6388,#6393,#1036,.F.);
#7810=EDGE_CURVE('',#6389,#6394,#1037,.T.);
#7811=EDGE_CURVE('',#6395,#6394,#5720,.T.);
#7812=EDGE_CURVE('',#6385,#6395,#1038,.F.);
#7813=EDGE_CURVE('',#6373,#6386,#5721,.T.);
#7814=EDGE_CURVE('',#6376,#6396,#1039,.T.);
#7815=EDGE_CURVE('',#6397,#6396,#5722,.T.);
#7816=EDGE_CURVE('',#6367,#6397,#1040,.F.);
#7817=EDGE_CURVE('',#6398,#6398,#5723,.T.);
#7818=EDGE_CURVE('',#6398,#6300,#3604,.T.);
#7819=EDGE_CURVE('',#6399,#6400,#5724,.T.);
#7820=EDGE_CURVE('',#6401,#6399,#3605,.T.);
#7821=EDGE_CURVE('',#6402,#6401,#5725,.T.);
#7822=EDGE_CURVE('',#6403,#6402,#3606,.T.);
#7823=EDGE_CURVE('',#6404,#6403,#5726,.T.);
#7824=EDGE_CURVE('',#6405,#6404,#3607,.T.);
#7825=EDGE_CURVE('',#6406,#6405,#5727,.T.);
#7826=EDGE_CURVE('',#6400,#6406,#3608,.T.);
#7827=EDGE_CURVE('',#6407,#6407,#5728,.T.);
#7828=EDGE_CURVE('',#6408,#6408,#5729,.T.);
#7829=EDGE_CURVE('',#6407,#6285,#3609,.T.);
#7830=EDGE_CURVE('',#6391,#6404,#1041,.F.);
#7831=EDGE_CURVE('',#6403,#6392,#1042,.T.);
#7832=EDGE_CURVE('',#6402,#6409,#5730,.T.);
#7833=EDGE_CURVE('',#6409,#6392,#3610,.T.);
#7834=EDGE_CURVE('',#6401,#6410,#5731,.T.);
#7835=EDGE_CURVE('',#6410,#6409,#5732,.T.);
#7836=EDGE_CURVE('',#6399,#6357,#1043,.F.);
#7837=EDGE_CURVE('',#6357,#6410,#3611,.T.);
#7838=EDGE_CURVE('',#6400,#6358,#1044,.T.);
#7839=EDGE_CURVE('',#6411,#6406,#5733,.T.);
#7840=EDGE_CURVE('',#6405,#6412,#5734,.T.);
#7841=EDGE_CURVE('',#6412,#6411,#5735,.T.);
#7842=EDGE_CURVE('',#6391,#6412,#3612,.T.);
#7843=EDGE_CURVE('',#6411,#6358,#3613,.T.);
#7844=EDGE_CURVE('',#6412,#6413,#3614,.T.);
#7845=EDGE_CURVE('',#6414,#6413,#5736,.T.);
#7846=EDGE_CURVE('',#6411,#6414,#3615,.T.);
#7847=EDGE_CURVE('',#6413,#6390,#3616,.T.);
#7848=EDGE_CURVE('',#6379,#6378,#5737,.T.);
#7849=EDGE_CURVE('',#6415,#6284,#5738,.T.);
#7850=EDGE_CURVE('',#6393,#6415,#3617,.T.);
#7851=EDGE_CURVE('',#6416,#6280,#5739,.T.);
#7852=EDGE_CURVE('',#6415,#6416,#5740,.T.);
#7853=EDGE_CURVE('',#6416,#6356,#3618,.T.);
#7854=EDGE_CURVE('',#6410,#6416,#3619,.T.);
#7855=EDGE_CURVE('',#6409,#6415,#3620,.T.);
#7856=EDGE_CURVE('',#6343,#6342,#5741,.T.);
#7857=EDGE_CURVE('',#6414,#6294,#5742,.T.);
#7858=EDGE_CURVE('',#6359,#6414,#3621,.T.);
#7859=EDGE_CURVE('',#6413,#6296,#5743,.T.);
#7860=EDGE_CURVE('',#6417,#6417,#5744,.T.);
#7861=EDGE_CURVE('',#6417,#6418,#5745,.T.);
#7862=EDGE_CURVE('',#6418,#6418,#5746,.T.);
#7863=EDGE_CURVE('',#6408,#6417,#3622,.T.);
#7864=EDGE_CURVE('',#6395,#6419,#3623,.T.);
#7865=EDGE_CURVE('',#6419,#6382,#5747,.T.);
#7866=EDGE_CURVE('',#6420,#6334,#5748,.T.);
#7867=EDGE_CURVE('',#6334,#6382,#5749,.T.);
#7868=EDGE_CURVE('',#6419,#6420,#5750,.T.);
#7869=EDGE_CURVE('',#6420,#6394,#3624,.T.);
#7870=EDGE_CURVE('',#6369,#6421,#5751,.T.);
#7871=EDGE_CURVE('',#6421,#6422,#5752,.T.);
#7872=EDGE_CURVE('',#6422,#6377,#5753,.T.);
#7873=EDGE_CURVE('',#6377,#6369,#5754,.T.);
#7874=EDGE_CURVE('',#6422,#6396,#3625,.T.);
#7875=EDGE_CURVE('',#6397,#6421,#3626,.T.);
#7876=EDGE_CURVE('',#6361,#6423,#3627,.T.);
#7877=EDGE_CURVE('',#6423,#6346,#5755,.T.);
#7878=EDGE_CURVE('',#6424,#6372,#5756,.T.);
#7879=EDGE_CURVE('',#6372,#6346,#5757,.T.);
#7880=EDGE_CURVE('',#6423,#6424,#5758,.T.);
#7881=EDGE_CURVE('',#6424,#6360,#3628,.T.);
#7882=EDGE_CURVE('',#6363,#6425,#3629,.T.);
#7883=EDGE_CURVE('',#6425,#6331,#5759,.T.);
#7884=EDGE_CURVE('',#6426,#6341,#5760,.T.);
#7885=EDGE_CURVE('',#6341,#6331,#5761,.T.);
#7886=EDGE_CURVE('',#6425,#6426,#5762,.T.);
#7887=EDGE_CURVE('',#6426,#6362,#3630,.T.);
#7888=EDGE_CURVE('',#6308,#6348,#5763,.T.);
#7889=EDGE_CURVE('',#6347,#6307,#5764,.T.);
#7890=EDGE_CURVE('',#6371,#6309,#5765,.T.);
#7891=EDGE_CURVE('',#6347,#6371,#5766,.T.);
#7892=EDGE_CURVE('',#6370,#6310,#5767,.T.);
#7893=EDGE_CURVE('',#6384,#6311,#5768,.T.);
#7894=EDGE_CURVE('',#6370,#6384,#5769,.T.);
#7895=EDGE_CURVE('',#6383,#6312,#5770,.T.);
#7896=EDGE_CURVE('',#6333,#6313,#5771,.T.);
#7897=EDGE_CURVE('',#6383,#6333,#5772,.T.);
#7898=EDGE_CURVE('',#6332,#6314,#5773,.T.);
#7899=EDGE_CURVE('',#6332,#6348,#5774,.T.);
#7900=EDGE_CURVE('',#6317,#6427,#5775,.T.);
#7901=EDGE_CURVE('',#6427,#6428,#5776,.T.);
#7902=EDGE_CURVE('',#6428,#6427,#5777,.T.);
#7903=EDGE_CURVE('',#6429,#6429,#5778,.T.);
#7904=EDGE_CURVE('',#6429,#6428,#3631,.T.);
#7905=EDGE_CURVE('',#6430,#6431,#1045,.T.);
#7906=EDGE_CURVE('',#6432,#6430,#1046,.T.);
#7907=EDGE_CURVE('',#6433,#6432,#1047,.T.);
#7908=EDGE_CURVE('',#6431,#6433,#1048,.T.);
#7909=EDGE_CURVE('',#6434,#6435,#1049,.T.);
#7910=EDGE_CURVE('',#6436,#6434,#1050,.T.);
#7911=EDGE_CURVE('',#6437,#6436,#1051,.T.);
#7912=EDGE_CURVE('',#6435,#6437,#1052,.T.);
#7913=EDGE_CURVE('',#6432,#6303,#5779,.T.);
#7914=EDGE_CURVE('',#6433,#6303,#1053,.F.);
#7915=EDGE_CURVE('',#6430,#6304,#5780,.T.);
#7916=EDGE_CURVE('',#6304,#6431,#1054,.F.);
#7917=EDGE_CURVE('',#6436,#6438,#5781,.T.);
#7918=EDGE_CURVE('',#6437,#6438,#1055,.F.);
#7919=EDGE_CURVE('',#6434,#6439,#5782,.T.);
#7920=EDGE_CURVE('',#6438,#6439,#5783,.T.);
#7921=EDGE_CURVE('',#6439,#6435,#1056,.F.);
#7922=EDGE_CURVE('',#6438,#6440,#1057,.T.);
#7923=EDGE_CURVE('',#6440,#6439,#1058,.T.);
#7924=EDGE_CURVE('',#6276,#6440,#3632,.T.);
#7925=EDGE_CURVE('',#6441,#6441,#5784,.T.);
#7926=EDGE_CURVE('',#6441,#6442,#3633,.T.);
#7927=EDGE_CURVE('',#6442,#6442,#5785,.T.);
#7928=EDGE_CURVE('',#6443,#6443,#5786,.T.);
#7929=EDGE_CURVE('',#6443,#6444,#3634,.T.);
#7930=EDGE_CURVE('',#6444,#6444,#5787,.T.);
#7931=EDGE_CURVE('',#6445,#6445,#5788,.T.);
#7932=EDGE_CURVE('',#6445,#6446,#3635,.T.);
#7933=EDGE_CURVE('',#6446,#6446,#5789,.T.);
#9799=ORIENTED_EDGE('',*,*,#7648,.T.);
#9800=ORIENTED_EDGE('',*,*,#7649,.T.);
#9801=ORIENTED_EDGE('',*,*,#7650,.T.);
#9802=ORIENTED_EDGE('',*,*,#7649,.F.);
#9803=ORIENTED_EDGE('',*,*,#7650,.F.);
#9804=ORIENTED_EDGE('',*,*,#7651,.T.);
#9805=ORIENTED_EDGE('',*,*,#7652,.F.);
#9806=ORIENTED_EDGE('',*,*,#7653,.F.);
#9807=ORIENTED_EDGE('',*,*,#7654,.F.);
#9808=ORIENTED_EDGE('',*,*,#7651,.F.);
#9809=ORIENTED_EDGE('',*,*,#7648,.F.);
#9810=ORIENTED_EDGE('',*,*,#7655,.T.);
#9811=ORIENTED_EDGE('',*,*,#7656,.T.);
#9812=ORIENTED_EDGE('',*,*,#7657,.T.);
#9813=ORIENTED_EDGE('',*,*,#7658,.T.);
#9814=ORIENTED_EDGE('',*,*,#7657,.F.);
#9815=ORIENTED_EDGE('',*,*,#7659,.F.);
#9816=ORIENTED_EDGE('',*,*,#7660,.F.);
#9817=ORIENTED_EDGE('',*,*,#7661,.T.);
#9818=ORIENTED_EDGE('',*,*,#7662,.F.);
#9819=ORIENTED_EDGE('',*,*,#7663,.F.);
#9820=ORIENTED_EDGE('',*,*,#7664,.F.);
#9821=ORIENTED_EDGE('',*,*,#7656,.F.);
#9822=ORIENTED_EDGE('',*,*,#7665,.F.);
#9823=ORIENTED_EDGE('',*,*,#7666,.T.);
#9824=ORIENTED_EDGE('',*,*,#7658,.F.);
#9825=ORIENTED_EDGE('',*,*,#7666,.F.);
#9826=ORIENTED_EDGE('',*,*,#7667,.T.);
#9827=ORIENTED_EDGE('',*,*,#7668,.T.);
#9828=ORIENTED_EDGE('',*,*,#7669,.T.);
#9829=ORIENTED_EDGE('',*,*,#7668,.F.);
#9830=ORIENTED_EDGE('',*,*,#7667,.F.);
#9831=ORIENTED_EDGE('',*,*,#7670,.F.);
#9832=ORIENTED_EDGE('',*,*,#7669,.F.);
#9833=ORIENTED_EDGE('',*,*,#7671,.T.);
#9834=ORIENTED_EDGE('',*,*,#7672,.F.);
#9835=ORIENTED_EDGE('',*,*,#7673,.F.);
#9836=ORIENTED_EDGE('',*,*,#7674,.F.);
#9837=ORIENTED_EDGE('',*,*,#7671,.F.);
#9838=ORIENTED_EDGE('',*,*,#7675,.T.);
#9839=ORIENTED_EDGE('',*,*,#7676,.T.);
#9840=ORIENTED_EDGE('',*,*,#7677,.T.);
#9841=ORIENTED_EDGE('',*,*,#7676,.F.);
#9842=ORIENTED_EDGE('',*,*,#7678,.F.);
#9843=ORIENTED_EDGE('',*,*,#7679,.F.);
#9844=ORIENTED_EDGE('',*,*,#7680,.F.);
#9845=ORIENTED_EDGE('',*,*,#7681,.F.);
#9846=ORIENTED_EDGE('',*,*,#7682,.T.);
#9847=ORIENTED_EDGE('',*,*,#7683,.F.);
#9848=ORIENTED_EDGE('',*,*,#7675,.F.);
#9849=ORIENTED_EDGE('',*,*,#7684,.F.);
#9850=ORIENTED_EDGE('',*,*,#7685,.T.);
#9851=ORIENTED_EDGE('',*,*,#7677,.F.);
#9852=ORIENTED_EDGE('',*,*,#7685,.F.);
#9853=ORIENTED_EDGE('',*,*,#7670,.T.);
#9854=ORIENTED_EDGE('',*,*,#7686,.T.);
#9855=ORIENTED_EDGE('',*,*,#7687,.T.);
#9856=ORIENTED_EDGE('',*,*,#7686,.F.);
#9857=ORIENTED_EDGE('',*,*,#7687,.F.);
#9858=ORIENTED_EDGE('',*,*,#7688,.T.);
#9859=ORIENTED_EDGE('',*,*,#7689,.F.);
#9860=ORIENTED_EDGE('',*,*,#7690,.T.);
#9861=ORIENTED_EDGE('',*,*,#7691,.F.);
#9862=ORIENTED_EDGE('',*,*,#7688,.F.);
#9863=ORIENTED_EDGE('',*,*,#7692,.T.);
#9864=ORIENTED_EDGE('',*,*,#7693,.T.);
#9865=ORIENTED_EDGE('',*,*,#7694,.T.);
#9866=ORIENTED_EDGE('',*,*,#7693,.F.);
#9867=ORIENTED_EDGE('',*,*,#7695,.F.);
#9868=ORIENTED_EDGE('',*,*,#7696,.F.);
#9869=ORIENTED_EDGE('',*,*,#7697,.F.);
#9870=ORIENTED_EDGE('',*,*,#7698,.F.);
#9871=ORIENTED_EDGE('',*,*,#7699,.F.);
#9872=ORIENTED_EDGE('',*,*,#7700,.F.);
#9873=ORIENTED_EDGE('',*,*,#7701,.F.);
#9874=ORIENTED_EDGE('',*,*,#7702,.F.);
#9875=ORIENTED_EDGE('',*,*,#7703,.F.);
#9876=ORIENTED_EDGE('',*,*,#7704,.F.);
#9877=ORIENTED_EDGE('',*,*,#7705,.F.);
#9878=ORIENTED_EDGE('',*,*,#7706,.F.);
#9879=ORIENTED_EDGE('',*,*,#7692,.F.);
#9880=ORIENTED_EDGE('',*,*,#7694,.F.);
#9881=ORIENTED_EDGE('',*,*,#7707,.T.);
#9882=ORIENTED_EDGE('',*,*,#7708,.T.);
#9883=ORIENTED_EDGE('',*,*,#7707,.F.);
#9884=ORIENTED_EDGE('',*,*,#7703,.T.);
#9885=ORIENTED_EDGE('',*,*,#7709,.T.);
#9886=ORIENTED_EDGE('',*,*,#7710,.T.);
#9887=ORIENTED_EDGE('',*,*,#7709,.F.);
#9888=ORIENTED_EDGE('',*,*,#7710,.F.);
#9889=ORIENTED_EDGE('',*,*,#7711,.T.);
#9890=ORIENTED_EDGE('',*,*,#7712,.T.);
#9891=ORIENTED_EDGE('',*,*,#7711,.F.);
#9892=ORIENTED_EDGE('',*,*,#7706,.T.);
#9893=ORIENTED_EDGE('',*,*,#7713,.T.);
#9894=ORIENTED_EDGE('',*,*,#7714,.T.);
#9895=ORIENTED_EDGE('',*,*,#7713,.F.);
#9896=ORIENTED_EDGE('',*,*,#7714,.F.);
#9897=ORIENTED_EDGE('',*,*,#7715,.T.);
#9898=ORIENTED_EDGE('',*,*,#7716,.T.);
#9899=ORIENTED_EDGE('',*,*,#7715,.F.);
#9900=ORIENTED_EDGE('',*,*,#7704,.T.);
#9901=ORIENTED_EDGE('',*,*,#7717,.T.);
#9902=ORIENTED_EDGE('',*,*,#7718,.T.);
#9903=ORIENTED_EDGE('',*,*,#7717,.F.);
#9904=ORIENTED_EDGE('',*,*,#7718,.F.);
#9905=ORIENTED_EDGE('',*,*,#7719,.T.);
#9906=ORIENTED_EDGE('',*,*,#7720,.T.);
#9907=ORIENTED_EDGE('',*,*,#7719,.F.);
#9908=ORIENTED_EDGE('',*,*,#7660,.T.);
#9909=ORIENTED_EDGE('',*,*,#7721,.T.);
#9910=ORIENTED_EDGE('',*,*,#7722,.T.);
#9911=ORIENTED_EDGE('',*,*,#7723,.T.);
#9912=ORIENTED_EDGE('',*,*,#7724,.T.);
#9913=ORIENTED_EDGE('',*,*,#7725,.T.);
#9914=ORIENTED_EDGE('',*,*,#7726,.T.);
#9915=ORIENTED_EDGE('',*,*,#7727,.T.);
#9916=ORIENTED_EDGE('',*,*,#7723,.F.);
#9917=ORIENTED_EDGE('',*,*,#7727,.F.);
#9918=ORIENTED_EDGE('',*,*,#7728,.F.);
#9919=ORIENTED_EDGE('',*,*,#7729,.T.);
#9920=ORIENTED_EDGE('',*,*,#7730,.F.);
#9921=ORIENTED_EDGE('',*,*,#7731,.F.);
#9922=ORIENTED_EDGE('',*,*,#7732,.F.);
#9923=ORIENTED_EDGE('',*,*,#7733,.F.);
#9924=ORIENTED_EDGE('',*,*,#7734,.F.);
#9925=ORIENTED_EDGE('',*,*,#7661,.F.);
#9926=ORIENTED_EDGE('',*,*,#7724,.F.);
#9927=ORIENTED_EDGE('',*,*,#7735,.T.);
#9928=ORIENTED_EDGE('',*,*,#7736,.T.);
#9929=ORIENTED_EDGE('',*,*,#7737,.T.);
#9930=ORIENTED_EDGE('',*,*,#7738,.T.);
#9931=ORIENTED_EDGE('',*,*,#7739,.F.);
#9932=ORIENTED_EDGE('',*,*,#7736,.F.);
#9933=ORIENTED_EDGE('',*,*,#7740,.F.);
#9934=ORIENTED_EDGE('',*,*,#7741,.F.);
#9935=ORIENTED_EDGE('',*,*,#7742,.F.);
#9936=ORIENTED_EDGE('',*,*,#7743,.F.);
#9937=ORIENTED_EDGE('',*,*,#7744,.F.);
#9938=ORIENTED_EDGE('',*,*,#7745,.T.);
#9939=ORIENTED_EDGE('',*,*,#7652,.T.);
#9940=ORIENTED_EDGE('',*,*,#7654,.T.);
#9941=ORIENTED_EDGE('',*,*,#7746,.T.);
#9942=ORIENTED_EDGE('',*,*,#7747,.F.);
#9943=ORIENTED_EDGE('',*,*,#7748,.F.);
#9944=ORIENTED_EDGE('',*,*,#7749,.T.);
#9945=ORIENTED_EDGE('',*,*,#7743,.T.);
#9946=ORIENTED_EDGE('',*,*,#7750,.T.);
#9947=ORIENTED_EDGE('',*,*,#7751,.T.);
#9948=ORIENTED_EDGE('',*,*,#7752,.T.);
#9949=ORIENTED_EDGE('',*,*,#7753,.T.);
#9950=ORIENTED_EDGE('',*,*,#7683,.T.);
#9951=ORIENTED_EDGE('',*,*,#7754,.T.);
#9952=ORIENTED_EDGE('',*,*,#7755,.T.);
#9953=ORIENTED_EDGE('',*,*,#7756,.T.);
#9954=ORIENTED_EDGE('',*,*,#7757,.T.);
#9955=ORIENTED_EDGE('',*,*,#7758,.T.);
#9956=ORIENTED_EDGE('',*,*,#7755,.F.);
#9957=ORIENTED_EDGE('',*,*,#7722,.F.);
#9958=ORIENTED_EDGE('',*,*,#7759,.F.);
#9959=ORIENTED_EDGE('',*,*,#7760,.F.);
#9960=ORIENTED_EDGE('',*,*,#7761,.F.);
#9961=ORIENTED_EDGE('',*,*,#7762,.T.);
#9962=ORIENTED_EDGE('',*,*,#7763,.F.);
#9963=ORIENTED_EDGE('',*,*,#7752,.F.);
#9964=ORIENTED_EDGE('',*,*,#7758,.F.);
#9965=ORIENTED_EDGE('',*,*,#7764,.T.);
#9966=ORIENTED_EDGE('',*,*,#7765,.F.);
#9967=ORIENTED_EDGE('',*,*,#7766,.F.);
#9968=ORIENTED_EDGE('',*,*,#7751,.F.);
#9969=ORIENTED_EDGE('',*,*,#7767,.F.);
#9970=ORIENTED_EDGE('',*,*,#7738,.F.);
#9971=ORIENTED_EDGE('',*,*,#7768,.T.);
#9972=ORIENTED_EDGE('',*,*,#7769,.F.);
#9973=ORIENTED_EDGE('',*,*,#7770,.F.);
#9974=ORIENTED_EDGE('',*,*,#7725,.F.);
#9975=ORIENTED_EDGE('',*,*,#7681,.T.);
#9976=ORIENTED_EDGE('',*,*,#7771,.T.);
#9977=ORIENTED_EDGE('',*,*,#7772,.T.);
#9978=ORIENTED_EDGE('',*,*,#7773,.T.);
#9979=ORIENTED_EDGE('',*,*,#7774,.T.);
#9980=ORIENTED_EDGE('',*,*,#7775,.T.);
#9981=ORIENTED_EDGE('',*,*,#7776,.T.);
#9982=ORIENTED_EDGE('',*,*,#7777,.T.);
#9983=ORIENTED_EDGE('',*,*,#7773,.F.);
#9984=ORIENTED_EDGE('',*,*,#7756,.F.);
#9985=ORIENTED_EDGE('',*,*,#7754,.F.);
#9986=ORIENTED_EDGE('',*,*,#7682,.F.);
#9987=ORIENTED_EDGE('',*,*,#7774,.F.);
#9988=ORIENTED_EDGE('',*,*,#7777,.F.);
#9989=ORIENTED_EDGE('',*,*,#7778,.F.);
#9990=ORIENTED_EDGE('',*,*,#7779,.T.);
#9991=ORIENTED_EDGE('',*,*,#7780,.F.);
#9992=ORIENTED_EDGE('',*,*,#7781,.F.);
#9993=ORIENTED_EDGE('',*,*,#7782,.F.);
#9994=ORIENTED_EDGE('',*,*,#7783,.T.);
#9995=ORIENTED_EDGE('',*,*,#7784,.T.);
#9996=ORIENTED_EDGE('',*,*,#7785,.T.);
#9997=ORIENTED_EDGE('',*,*,#7786,.T.);
#9998=ORIENTED_EDGE('',*,*,#7787,.F.);
#9999=ORIENTED_EDGE('',*,*,#7784,.F.);
#10000=ORIENTED_EDGE('',*,*,#7788,.F.);
#10001=ORIENTED_EDGE('',*,*,#7789,.F.);
#10002=ORIENTED_EDGE('',*,*,#7790,.F.);
#10003=ORIENTED_EDGE('',*,*,#7791,.F.);
#10004=ORIENTED_EDGE('',*,*,#7792,.F.);
#10005=ORIENTED_EDGE('',*,*,#7793,.T.);
#10006=ORIENTED_EDGE('',*,*,#7794,.F.);
#10007=ORIENTED_EDGE('',*,*,#7795,.F.);
#10008=ORIENTED_EDGE('',*,*,#7672,.T.);
#10009=ORIENTED_EDGE('',*,*,#7674,.T.);
#10010=ORIENTED_EDGE('',*,*,#7796,.F.);
#10011=ORIENTED_EDGE('',*,*,#7797,.T.);
#10012=ORIENTED_EDGE('',*,*,#7791,.T.);
#10013=ORIENTED_EDGE('',*,*,#7798,.T.);
#10014=ORIENTED_EDGE('',*,*,#7799,.T.);
#10015=ORIENTED_EDGE('',*,*,#7800,.T.);
#10016=ORIENTED_EDGE('',*,*,#7801,.T.);
#10017=ORIENTED_EDGE('',*,*,#7662,.T.);
#10018=ORIENTED_EDGE('',*,*,#7734,.T.);
#10019=ORIENTED_EDGE('',*,*,#7802,.T.);
#10020=ORIENTED_EDGE('',*,*,#7733,.T.);
#10021=ORIENTED_EDGE('',*,*,#7803,.T.);
#10022=ORIENTED_EDGE('',*,*,#7804,.T.);
#10023=ORIENTED_EDGE('',*,*,#7802,.F.);
#10024=ORIENTED_EDGE('',*,*,#7772,.F.);
#10025=ORIENTED_EDGE('',*,*,#7805,.F.);
#10026=ORIENTED_EDGE('',*,*,#7806,.F.);
#10027=ORIENTED_EDGE('',*,*,#7807,.F.);
#10028=ORIENTED_EDGE('',*,*,#7808,.T.);
#10029=ORIENTED_EDGE('',*,*,#7809,.F.);
#10030=ORIENTED_EDGE('',*,*,#7800,.F.);
#10031=ORIENTED_EDGE('',*,*,#7804,.F.);
#10032=ORIENTED_EDGE('',*,*,#7810,.T.);
#10033=ORIENTED_EDGE('',*,*,#7811,.F.);
#10034=ORIENTED_EDGE('',*,*,#7812,.F.);
#10035=ORIENTED_EDGE('',*,*,#7799,.F.);
#10036=ORIENTED_EDGE('',*,*,#7813,.F.);
#10037=ORIENTED_EDGE('',*,*,#7786,.F.);
#10038=ORIENTED_EDGE('',*,*,#7814,.T.);
#10039=ORIENTED_EDGE('',*,*,#7815,.F.);
#10040=ORIENTED_EDGE('',*,*,#7816,.F.);
#10041=ORIENTED_EDGE('',*,*,#7775,.F.);
#10042=ORIENTED_EDGE('',*,*,#7817,.T.);
#10043=ORIENTED_EDGE('',*,*,#7818,.T.);
#10044=ORIENTED_EDGE('',*,*,#7684,.T.);
#10045=ORIENTED_EDGE('',*,*,#7818,.F.);
#10046=ORIENTED_EDGE('',*,*,#7819,.F.);
#10047=ORIENTED_EDGE('',*,*,#7820,.F.);
#10048=ORIENTED_EDGE('',*,*,#7821,.F.);
#10049=ORIENTED_EDGE('',*,*,#7822,.F.);
#10050=ORIENTED_EDGE('',*,*,#7823,.F.);
#10051=ORIENTED_EDGE('',*,*,#7824,.F.);
#10052=ORIENTED_EDGE('',*,*,#7825,.F.);
#10053=ORIENTED_EDGE('',*,*,#7826,.F.);
#10054=ORIENTED_EDGE('',*,*,#7827,.F.);
#10055=ORIENTED_EDGE('',*,*,#7828,.T.);
#10056=ORIENTED_EDGE('',*,*,#7817,.F.);
#10057=ORIENTED_EDGE('',*,*,#7827,.T.);
#10058=ORIENTED_EDGE('',*,*,#7829,.T.);
#10059=ORIENTED_EDGE('',*,*,#7665,.T.);
#10060=ORIENTED_EDGE('',*,*,#7829,.F.);
#10061=ORIENTED_EDGE('',*,*,#7807,.T.);
#10062=ORIENTED_EDGE('',*,*,#7830,.T.);
#10063=ORIENTED_EDGE('',*,*,#7823,.T.);
#10064=ORIENTED_EDGE('',*,*,#7831,.T.);
#10065=ORIENTED_EDGE('',*,*,#7822,.T.);
#10066=ORIENTED_EDGE('',*,*,#7832,.T.);
#10067=ORIENTED_EDGE('',*,*,#7833,.T.);
#10068=ORIENTED_EDGE('',*,*,#7831,.F.);
#10069=ORIENTED_EDGE('',*,*,#7834,.T.);
#10070=ORIENTED_EDGE('',*,*,#7835,.T.);
#10071=ORIENTED_EDGE('',*,*,#7832,.F.);
#10072=ORIENTED_EDGE('',*,*,#7821,.T.);
#10073=ORIENTED_EDGE('',*,*,#7836,.T.);
#10074=ORIENTED_EDGE('',*,*,#7837,.T.);
#10075=ORIENTED_EDGE('',*,*,#7834,.F.);
#10076=ORIENTED_EDGE('',*,*,#7820,.T.);
#10077=ORIENTED_EDGE('',*,*,#7761,.T.);
#10078=ORIENTED_EDGE('',*,*,#7836,.F.);
#10079=ORIENTED_EDGE('',*,*,#7819,.T.);
#10080=ORIENTED_EDGE('',*,*,#7838,.T.);
#10081=ORIENTED_EDGE('',*,*,#7839,.T.);
#10082=ORIENTED_EDGE('',*,*,#7825,.T.);
#10083=ORIENTED_EDGE('',*,*,#7840,.T.);
#10084=ORIENTED_EDGE('',*,*,#7841,.T.);
#10085=ORIENTED_EDGE('',*,*,#7842,.T.);
#10086=ORIENTED_EDGE('',*,*,#7840,.F.);
#10087=ORIENTED_EDGE('',*,*,#7824,.T.);
#10088=ORIENTED_EDGE('',*,*,#7830,.F.);
#10089=ORIENTED_EDGE('',*,*,#7826,.T.);
#10090=ORIENTED_EDGE('',*,*,#7839,.F.);
#10091=ORIENTED_EDGE('',*,*,#7843,.T.);
#10092=ORIENTED_EDGE('',*,*,#7838,.F.);
#10093=ORIENTED_EDGE('',*,*,#7841,.F.);
#10094=ORIENTED_EDGE('',*,*,#7844,.T.);
#10095=ORIENTED_EDGE('',*,*,#7845,.F.);
#10096=ORIENTED_EDGE('',*,*,#7846,.F.);
#10097=ORIENTED_EDGE('',*,*,#7842,.F.);
#10098=ORIENTED_EDGE('',*,*,#7806,.T.);
#10099=ORIENTED_EDGE('',*,*,#7847,.F.);
#10100=ORIENTED_EDGE('',*,*,#7844,.F.);
#10101=ORIENTED_EDGE('',*,*,#7788,.T.);
#10102=ORIENTED_EDGE('',*,*,#7783,.F.);
#10103=ORIENTED_EDGE('',*,*,#7813,.T.);
#10104=ORIENTED_EDGE('',*,*,#7798,.F.);
#10105=ORIENTED_EDGE('',*,*,#7790,.T.);
#10106=ORIENTED_EDGE('',*,*,#7848,.T.);
#10107=ORIENTED_EDGE('',*,*,#7849,.T.);
#10108=ORIENTED_EDGE('',*,*,#7663,.T.);
#10109=ORIENTED_EDGE('',*,*,#7801,.F.);
#10110=ORIENTED_EDGE('',*,*,#7809,.T.);
#10111=ORIENTED_EDGE('',*,*,#7850,.T.);
#10112=ORIENTED_EDGE('',*,*,#7851,.T.);
#10113=ORIENTED_EDGE('',*,*,#7664,.T.);
#10114=ORIENTED_EDGE('',*,*,#7849,.F.);
#10115=ORIENTED_EDGE('',*,*,#7852,.T.);
#10116=ORIENTED_EDGE('',*,*,#7759,.T.);
#10117=ORIENTED_EDGE('',*,*,#7721,.F.);
#10118=ORIENTED_EDGE('',*,*,#7659,.T.);
#10119=ORIENTED_EDGE('',*,*,#7851,.F.);
#10120=ORIENTED_EDGE('',*,*,#7853,.T.);
#10121=ORIENTED_EDGE('',*,*,#7837,.F.);
#10122=ORIENTED_EDGE('',*,*,#7760,.T.);
#10123=ORIENTED_EDGE('',*,*,#7853,.F.);
#10124=ORIENTED_EDGE('',*,*,#7854,.F.);
#10125=ORIENTED_EDGE('',*,*,#7835,.F.);
#10126=ORIENTED_EDGE('',*,*,#7854,.T.);
#10127=ORIENTED_EDGE('',*,*,#7852,.F.);
#10128=ORIENTED_EDGE('',*,*,#7855,.F.);
#10129=ORIENTED_EDGE('',*,*,#7833,.F.);
#10130=ORIENTED_EDGE('',*,*,#7855,.T.);
#10131=ORIENTED_EDGE('',*,*,#7850,.F.);
#10132=ORIENTED_EDGE('',*,*,#7808,.F.);
#10133=ORIENTED_EDGE('',*,*,#7740,.T.);
#10134=ORIENTED_EDGE('',*,*,#7735,.F.);
#10135=ORIENTED_EDGE('',*,*,#7767,.T.);
#10136=ORIENTED_EDGE('',*,*,#7750,.F.);
#10137=ORIENTED_EDGE('',*,*,#7742,.T.);
#10138=ORIENTED_EDGE('',*,*,#7856,.T.);
#10139=ORIENTED_EDGE('',*,*,#7857,.T.);
#10140=ORIENTED_EDGE('',*,*,#7678,.T.);
#10141=ORIENTED_EDGE('',*,*,#7753,.F.);
#10142=ORIENTED_EDGE('',*,*,#7763,.T.);
#10143=ORIENTED_EDGE('',*,*,#7858,.T.);
#10144=ORIENTED_EDGE('',*,*,#7859,.T.);
#10145=ORIENTED_EDGE('',*,*,#7679,.T.);
#10146=ORIENTED_EDGE('',*,*,#7857,.F.);
#10147=ORIENTED_EDGE('',*,*,#7845,.T.);
#10148=ORIENTED_EDGE('',*,*,#7805,.T.);
#10149=ORIENTED_EDGE('',*,*,#7771,.F.);
#10150=ORIENTED_EDGE('',*,*,#7680,.T.);
#10151=ORIENTED_EDGE('',*,*,#7859,.F.);
#10152=ORIENTED_EDGE('',*,*,#7847,.T.);
#10153=ORIENTED_EDGE('',*,*,#7843,.F.);
#10154=ORIENTED_EDGE('',*,*,#7846,.T.);
#10155=ORIENTED_EDGE('',*,*,#7858,.F.);
#10156=ORIENTED_EDGE('',*,*,#7762,.F.);
#10157=ORIENTED_EDGE('',*,*,#7860,.T.);
#10158=ORIENTED_EDGE('',*,*,#7861,.T.);
#10159=ORIENTED_EDGE('',*,*,#7862,.T.);
#10160=ORIENTED_EDGE('',*,*,#7861,.F.);
#10161=ORIENTED_EDGE('',*,*,#7828,.F.);
#10162=ORIENTED_EDGE('',*,*,#7863,.T.);
#10163=ORIENTED_EDGE('',*,*,#7860,.F.);
#10164=ORIENTED_EDGE('',*,*,#7863,.F.);
#10165=ORIENTED_EDGE('',*,*,#7812,.T.);
#10166=ORIENTED_EDGE('',*,*,#7864,.T.);
#10167=ORIENTED_EDGE('',*,*,#7865,.T.);
#10168=ORIENTED_EDGE('',*,*,#7792,.T.);
#10169=ORIENTED_EDGE('',*,*,#7797,.F.);
#10170=ORIENTED_EDGE('',*,*,#7866,.T.);
#10171=ORIENTED_EDGE('',*,*,#7867,.T.);
#10172=ORIENTED_EDGE('',*,*,#7865,.F.);
#10173=ORIENTED_EDGE('',*,*,#7868,.T.);
#10174=ORIENTED_EDGE('',*,*,#7732,.T.);
#10175=ORIENTED_EDGE('',*,*,#7866,.F.);
#10176=ORIENTED_EDGE('',*,*,#7869,.T.);
#10177=ORIENTED_EDGE('',*,*,#7810,.F.);
#10178=ORIENTED_EDGE('',*,*,#7803,.F.);
#10179=ORIENTED_EDGE('',*,*,#7869,.F.);
#10180=ORIENTED_EDGE('',*,*,#7868,.F.);
#10181=ORIENTED_EDGE('',*,*,#7864,.F.);
#10182=ORIENTED_EDGE('',*,*,#7811,.T.);
#10183=ORIENTED_EDGE('',*,*,#7870,.T.);
#10184=ORIENTED_EDGE('',*,*,#7871,.T.);
#10185=ORIENTED_EDGE('',*,*,#7872,.T.);
#10186=ORIENTED_EDGE('',*,*,#7873,.T.);
#10187=ORIENTED_EDGE('',*,*,#7787,.T.);
#10188=ORIENTED_EDGE('',*,*,#7872,.F.);
#10189=ORIENTED_EDGE('',*,*,#7874,.T.);
#10190=ORIENTED_EDGE('',*,*,#7814,.F.);
#10191=ORIENTED_EDGE('',*,*,#7785,.F.);
#10192=ORIENTED_EDGE('',*,*,#7816,.T.);
#10193=ORIENTED_EDGE('',*,*,#7875,.T.);
#10194=ORIENTED_EDGE('',*,*,#7870,.F.);
#10195=ORIENTED_EDGE('',*,*,#7778,.T.);
#10196=ORIENTED_EDGE('',*,*,#7776,.F.);
#10197=ORIENTED_EDGE('',*,*,#7874,.F.);
#10198=ORIENTED_EDGE('',*,*,#7871,.F.);
#10199=ORIENTED_EDGE('',*,*,#7875,.F.);
#10200=ORIENTED_EDGE('',*,*,#7815,.T.);
#10201=ORIENTED_EDGE('',*,*,#7766,.T.);
#10202=ORIENTED_EDGE('',*,*,#7876,.T.);
#10203=ORIENTED_EDGE('',*,*,#7877,.T.);
#10204=ORIENTED_EDGE('',*,*,#7744,.T.);
#10205=ORIENTED_EDGE('',*,*,#7749,.F.);
#10206=ORIENTED_EDGE('',*,*,#7878,.T.);
#10207=ORIENTED_EDGE('',*,*,#7879,.T.);
#10208=ORIENTED_EDGE('',*,*,#7877,.F.);
#10209=ORIENTED_EDGE('',*,*,#7880,.T.);
#10210=ORIENTED_EDGE('',*,*,#7782,.T.);
#10211=ORIENTED_EDGE('',*,*,#7878,.F.);
#10212=ORIENTED_EDGE('',*,*,#7881,.T.);
#10213=ORIENTED_EDGE('',*,*,#7764,.F.);
#10214=ORIENTED_EDGE('',*,*,#7757,.F.);
#10215=ORIENTED_EDGE('',*,*,#7881,.F.);
#10216=ORIENTED_EDGE('',*,*,#7880,.F.);
#10217=ORIENTED_EDGE('',*,*,#7876,.F.);
#10218=ORIENTED_EDGE('',*,*,#7765,.T.);
#10219=ORIENTED_EDGE('',*,*,#7770,.T.);
#10220=ORIENTED_EDGE('',*,*,#7882,.T.);
#10221=ORIENTED_EDGE('',*,*,#7883,.T.);
#10222=ORIENTED_EDGE('',*,*,#7728,.T.);
#10223=ORIENTED_EDGE('',*,*,#7726,.F.);
#10224=ORIENTED_EDGE('',*,*,#7884,.T.);
#10225=ORIENTED_EDGE('',*,*,#7885,.T.);
#10226=ORIENTED_EDGE('',*,*,#7883,.F.);
#10227=ORIENTED_EDGE('',*,*,#7886,.T.);
#10228=ORIENTED_EDGE('',*,*,#7739,.T.);
#10229=ORIENTED_EDGE('',*,*,#7884,.F.);
#10230=ORIENTED_EDGE('',*,*,#7887,.T.);
#10231=ORIENTED_EDGE('',*,*,#7768,.F.);
#10232=ORIENTED_EDGE('',*,*,#7737,.F.);
#10233=ORIENTED_EDGE('',*,*,#7887,.F.);
#10234=ORIENTED_EDGE('',*,*,#7886,.F.);
#10235=ORIENTED_EDGE('',*,*,#7882,.F.);
#10236=ORIENTED_EDGE('',*,*,#7769,.T.);
#10237=ORIENTED_EDGE('',*,*,#7888,.T.);
#10238=ORIENTED_EDGE('',*,*,#7747,.T.);
#10239=ORIENTED_EDGE('',*,*,#7889,.T.);
#10240=ORIENTED_EDGE('',*,*,#7695,.T.);
#10241=ORIENTED_EDGE('',*,*,#7890,.T.);
#10242=ORIENTED_EDGE('',*,*,#7696,.T.);
#10243=ORIENTED_EDGE('',*,*,#7889,.F.);
#10244=ORIENTED_EDGE('',*,*,#7891,.T.);
#10245=ORIENTED_EDGE('',*,*,#7892,.T.);
#10246=ORIENTED_EDGE('',*,*,#7697,.T.);
#10247=ORIENTED_EDGE('',*,*,#7890,.F.);
#10248=ORIENTED_EDGE('',*,*,#7780,.T.);
#10249=ORIENTED_EDGE('',*,*,#7893,.T.);
#10250=ORIENTED_EDGE('',*,*,#7698,.T.);
#10251=ORIENTED_EDGE('',*,*,#7892,.F.);
#10252=ORIENTED_EDGE('',*,*,#7894,.T.);
#10253=ORIENTED_EDGE('',*,*,#7895,.T.);
#10254=ORIENTED_EDGE('',*,*,#7699,.T.);
#10255=ORIENTED_EDGE('',*,*,#7893,.F.);
#10256=ORIENTED_EDGE('',*,*,#7794,.T.);
#10257=ORIENTED_EDGE('',*,*,#7896,.T.);
#10258=ORIENTED_EDGE('',*,*,#7700,.T.);
#10259=ORIENTED_EDGE('',*,*,#7895,.F.);
#10260=ORIENTED_EDGE('',*,*,#7897,.T.);
#10261=ORIENTED_EDGE('',*,*,#7898,.T.);
#10262=ORIENTED_EDGE('',*,*,#7701,.T.);
#10263=ORIENTED_EDGE('',*,*,#7896,.F.);
#10264=ORIENTED_EDGE('',*,*,#7730,.T.);
#10265=ORIENTED_EDGE('',*,*,#7888,.F.);
#10266=ORIENTED_EDGE('',*,*,#7702,.T.);
#10267=ORIENTED_EDGE('',*,*,#7898,.F.);
#10268=ORIENTED_EDGE('',*,*,#7899,.T.);
#10269=ORIENTED_EDGE('',*,*,#7873,.F.);
#10270=ORIENTED_EDGE('',*,*,#7796,.T.);
#10271=ORIENTED_EDGE('',*,*,#7673,.T.);
#10272=ORIENTED_EDGE('',*,*,#7795,.T.);
#10273=ORIENTED_EDGE('',*,*,#7894,.F.);
#10274=ORIENTED_EDGE('',*,*,#7779,.F.);
#10275=ORIENTED_EDGE('',*,*,#7879,.F.);
#10276=ORIENTED_EDGE('',*,*,#7781,.T.);
#10277=ORIENTED_EDGE('',*,*,#7891,.F.);
#10278=ORIENTED_EDGE('',*,*,#7746,.F.);
#10279=ORIENTED_EDGE('',*,*,#7653,.T.);
#10280=ORIENTED_EDGE('',*,*,#7745,.F.);
#10281=ORIENTED_EDGE('',*,*,#7705,.T.);
#10282=ORIENTED_EDGE('',*,*,#7900,.T.);
#10283=ORIENTED_EDGE('',*,*,#7901,.T.);
#10284=ORIENTED_EDGE('',*,*,#7902,.T.);
#10285=ORIENTED_EDGE('',*,*,#7900,.F.);
#10286=ORIENTED_EDGE('',*,*,#7903,.F.);
#10287=ORIENTED_EDGE('',*,*,#7904,.T.);
#10288=ORIENTED_EDGE('',*,*,#7901,.F.);
#10289=ORIENTED_EDGE('',*,*,#7902,.F.);
#10290=ORIENTED_EDGE('',*,*,#7904,.F.);
#10291=ORIENTED_EDGE('',*,*,#7905,.F.);
#10292=ORIENTED_EDGE('',*,*,#7906,.F.);
#10293=ORIENTED_EDGE('',*,*,#7907,.F.);
#10294=ORIENTED_EDGE('',*,*,#7908,.F.);
#10295=ORIENTED_EDGE('',*,*,#7909,.F.);
#10296=ORIENTED_EDGE('',*,*,#7910,.F.);
#10297=ORIENTED_EDGE('',*,*,#7911,.F.);
#10298=ORIENTED_EDGE('',*,*,#7912,.F.);
#10299=ORIENTED_EDGE('',*,*,#7913,.T.);
#10300=ORIENTED_EDGE('',*,*,#7914,.F.);
#10301=ORIENTED_EDGE('',*,*,#7907,.T.);
#10302=ORIENTED_EDGE('',*,*,#7915,.T.);
#10303=ORIENTED_EDGE('',*,*,#7690,.F.);
#10304=ORIENTED_EDGE('',*,*,#7913,.F.);
#10305=ORIENTED_EDGE('',*,*,#7906,.T.);
#10306=ORIENTED_EDGE('',*,*,#7915,.F.);
#10307=ORIENTED_EDGE('',*,*,#7905,.T.);
#10308=ORIENTED_EDGE('',*,*,#7916,.F.);
#10309=ORIENTED_EDGE('',*,*,#7914,.T.);
#10310=ORIENTED_EDGE('',*,*,#7689,.T.);
#10311=ORIENTED_EDGE('',*,*,#7691,.T.);
#10312=ORIENTED_EDGE('',*,*,#7916,.T.);
#10313=ORIENTED_EDGE('',*,*,#7908,.T.);
#10314=ORIENTED_EDGE('',*,*,#7917,.T.);
#10315=ORIENTED_EDGE('',*,*,#7918,.F.);
#10316=ORIENTED_EDGE('',*,*,#7911,.T.);
#10317=ORIENTED_EDGE('',*,*,#7919,.T.);
#10318=ORIENTED_EDGE('',*,*,#7920,.F.);
#10319=ORIENTED_EDGE('',*,*,#7917,.F.);
#10320=ORIENTED_EDGE('',*,*,#7910,.T.);
#10321=ORIENTED_EDGE('',*,*,#7919,.F.);
#10322=ORIENTED_EDGE('',*,*,#7909,.T.);
#10323=ORIENTED_EDGE('',*,*,#7921,.F.);
#10324=ORIENTED_EDGE('',*,*,#7918,.T.);
#10325=ORIENTED_EDGE('',*,*,#7922,.T.);
#10326=ORIENTED_EDGE('',*,*,#7923,.T.);
#10327=ORIENTED_EDGE('',*,*,#7921,.T.);
#10328=ORIENTED_EDGE('',*,*,#7912,.T.);
#10329=ORIENTED_EDGE('',*,*,#7655,.F.);
#10330=ORIENTED_EDGE('',*,*,#7924,.T.);
#10331=ORIENTED_EDGE('',*,*,#7922,.F.);
#10332=ORIENTED_EDGE('',*,*,#7920,.T.);
#10333=ORIENTED_EDGE('',*,*,#7923,.F.);
#10334=ORIENTED_EDGE('',*,*,#7924,.F.);
#10335=ORIENTED_EDGE('',*,*,#7708,.F.);
#10336=ORIENTED_EDGE('',*,*,#7712,.F.);
#10337=ORIENTED_EDGE('',*,*,#7716,.F.);
#10338=ORIENTED_EDGE('',*,*,#7720,.F.);
#10339=ORIENTED_EDGE('',*,*,#7925,.F.);
#10340=ORIENTED_EDGE('',*,*,#7926,.T.);
#10341=ORIENTED_EDGE('',*,*,#7927,.T.);
#10342=ORIENTED_EDGE('',*,*,#7926,.F.);
#10343=ORIENTED_EDGE('',*,*,#7928,.T.);
#10344=ORIENTED_EDGE('',*,*,#7927,.F.);
#10345=ORIENTED_EDGE('',*,*,#7928,.F.);
#10346=ORIENTED_EDGE('',*,*,#7929,.T.);
#10347=ORIENTED_EDGE('',*,*,#7930,.T.);
#10348=ORIENTED_EDGE('',*,*,#7929,.F.);
#10349=ORIENTED_EDGE('',*,*,#7930,.F.);
#10350=ORIENTED_EDGE('',*,*,#7931,.T.);
#10351=ORIENTED_EDGE('',*,*,#7931,.F.);
#10352=ORIENTED_EDGE('',*,*,#7932,.T.);
#10353=ORIENTED_EDGE('',*,*,#7933,.T.);
#10354=ORIENTED_EDGE('',*,*,#7932,.F.);
#10355=ORIENTED_EDGE('',*,*,#7903,.T.);
#10356=ORIENTED_EDGE('',*,*,#7933,.F.);
#10357=ORIENTED_EDGE('',*,*,#7862,.F.);
#10358=ORIENTED_EDGE('',*,*,#7925,.T.);
#10359=ORIENTED_EDGE('',*,*,#7867,.F.);
#10360=ORIENTED_EDGE('',*,*,#7731,.T.);
#10361=ORIENTED_EDGE('',*,*,#7897,.F.);
#10362=ORIENTED_EDGE('',*,*,#7793,.F.);
#10363=ORIENTED_EDGE('',*,*,#7885,.F.);
#10364=ORIENTED_EDGE('',*,*,#7748,.T.);
#10365=ORIENTED_EDGE('',*,*,#7899,.F.);
#10366=ORIENTED_EDGE('',*,*,#7729,.F.);
#10367=ORIENTED_EDGE('',*,*,#7856,.F.);
#10368=ORIENTED_EDGE('',*,*,#7741,.T.);
#10369=ORIENTED_EDGE('',*,*,#7848,.F.);
#10370=ORIENTED_EDGE('',*,*,#7789,.T.);
#14101=CONICAL_SURFACE('',#15254,14.75,0.785398163397448);
#14102=CONICAL_SURFACE('',#15262,7.4,0.785398163397448);
#14103=CONICAL_SURFACE('',#15271,14.75,0.785398163397448);
#14104=CONICAL_SURFACE('',#15279,7.4,0.785398163397448);
#14105=CONICAL_SURFACE('',#15288,9.3,0.785398163397448);
#14106=CONICAL_SURFACE('',#15292,6.3,0.785398163397439);
#14107=CONICAL_SURFACE('',#15306,6.3,0.785398163397439);
#14108=CONICAL_SURFACE('',#15310,6.3,0.785398163397439);
#14109=CONICAL_SURFACE('',#15314,6.3,0.785398163397439);
#14110=CONICAL_SURFACE('',#15318,62.25,0.785398163397446);
#14111=CONICAL_SURFACE('',#15328,62.25,0.785398163397446);
#14112=CONICAL_SURFACE('',#15337,62.25,0.785398163397455);
#14113=CONICAL_SURFACE('',#15347,62.25,0.785398163397455);
#14114=CONICAL_SURFACE('',#15356,7.4,0.785398163397449);
#14115=CONICAL_SURFACE('',#15365,7.4,0.785398163397449);
#14184=ADVANCED_FACE('',(#1617),#14101,.T.);
#14185=ADVANCED_FACE('',(#1618),#1366,.T.);
#14186=ADVANCED_FACE('',(#1619,#417),#558,.F.);
#14187=ADVANCED_FACE('',(#1620),#14102,.F.);
#14188=ADVANCED_FACE('',(#1621,#418),#559,.T.);
#14189=ADVANCED_FACE('',(#1622),#1367,.F.);
#14190=ADVANCED_FACE('',(#1623),#14103,.T.);
#14191=ADVANCED_FACE('',(#1624,#419),#560,.T.);
#14192=ADVANCED_FACE('',(#1625),#1368,.T.);
#14193=ADVANCED_FACE('',(#1626),#14104,.F.);
#14194=ADVANCED_FACE('',(#1627,#420),#561,.T.);
#14195=ADVANCED_FACE('',(#1628),#1369,.F.);
#14196=ADVANCED_FACE('',(#1629),#14105,.F.);
#14197=ADVANCED_FACE('',(#1630),#1370,.F.);
#14198=ADVANCED_FACE('',(#1631),#14106,.F.);
#14199=ADVANCED_FACE('',(#1632,#421,#422,#423,#424,#425),#562,.T.);
#14200=ADVANCED_FACE('',(#1633),#1371,.F.);
#14201=ADVANCED_FACE('',(#1634),#14107,.F.);
#14202=ADVANCED_FACE('',(#1635),#1372,.F.);
#14203=ADVANCED_FACE('',(#1636),#14108,.F.);
#14204=ADVANCED_FACE('',(#1637),#1373,.F.);
#14205=ADVANCED_FACE('',(#1638),#14109,.F.);
#14206=ADVANCED_FACE('',(#1639),#1374,.F.);
#14207=ADVANCED_FACE('',(#1640),#14110,.T.);
#14208=ADVANCED_FACE('',(#1641),#563,.T.);
#14209=ADVANCED_FACE('',(#1642),#564,.T.);
#14210=ADVANCED_FACE('',(#1643),#565,.T.);
#14211=ADVANCED_FACE('',(#1644),#566,.T.);
#14212=ADVANCED_FACE('',(#1645),#567,.T.);
#14213=ADVANCED_FACE('',(#1646),#14111,.T.);
#14214=ADVANCED_FACE('',(#1647),#568,.T.);
#14215=ADVANCED_FACE('',(#1648),#1375,.T.);
#14216=ADVANCED_FACE('',(#1649),#14112,.T.);
#14217=ADVANCED_FACE('',(#1650),#569,.T.);
#14218=ADVANCED_FACE('',(#1651),#570,.T.);
#14219=ADVANCED_FACE('',(#1652),#571,.T.);
#14220=ADVANCED_FACE('',(#1653),#572,.T.);
#14221=ADVANCED_FACE('',(#1654),#573,.T.);
#14222=ADVANCED_FACE('',(#1655),#14113,.T.);
#14223=ADVANCED_FACE('',(#1656),#574,.T.);
#14224=ADVANCED_FACE('',(#1657),#1376,.T.);
#14225=ADVANCED_FACE('',(#1658),#14114,.F.);
#14226=ADVANCED_FACE('',(#1659,#426,#427,#428),#575,.F.);
#14227=ADVANCED_FACE('',(#1660),#14115,.F.);
#14228=ADVANCED_FACE('',(#1661),#256,.T.);
#14229=ADVANCED_FACE('',(#1662),#1377,.T.);
#14230=ADVANCED_FACE('',(#1663),#257,.T.);
#14231=ADVANCED_FACE('',(#1664),#1378,.T.);
#14232=ADVANCED_FACE('',(#1665),#258,.T.);
#14233=ADVANCED_FACE('',(#1666),#259,.T.);
#14234=ADVANCED_FACE('',(#1667),#1379,.T.);
#14235=ADVANCED_FACE('',(#1668),#1380,.T.);
#14236=ADVANCED_FACE('',(#1669),#1381,.T.);
#14237=ADVANCED_FACE('',(#1670),#576,.T.);
#14238=ADVANCED_FACE('',(#1671),#260,.T.);
#14239=ADVANCED_FACE('',(#1672),#1382,.T.);
#14240=ADVANCED_FACE('',(#1673),#261,.T.);
#14241=ADVANCED_FACE('',(#1674),#1383,.T.);
#14242=ADVANCED_FACE('',(#1675),#577,.T.);
#14243=ADVANCED_FACE('',(#1676),#1384,.T.);
#14244=ADVANCED_FACE('',(#1677),#578,.T.);
#14245=ADVANCED_FACE('',(#1678),#262,.T.);
#14246=ADVANCED_FACE('',(#1679),#1385,.T.);
#14247=ADVANCED_FACE('',(#1680),#263,.T.);
#14248=ADVANCED_FACE('',(#1681),#1386,.T.);
#14249=ADVANCED_FACE('',(#1682),#579,.T.);
#14250=ADVANCED_FACE('',(#1683),#264,.T.);
#14251=ADVANCED_FACE('',(#1684),#1387,.T.);
#14252=ADVANCED_FACE('',(#1685),#1388,.T.);
#14253=ADVANCED_FACE('',(#1686),#265,.T.);
#14254=ADVANCED_FACE('',(#1687),#1389,.T.);
#14255=ADVANCED_FACE('',(#1688),#580,.F.);
#14256=ADVANCED_FACE('',(#1689),#266,.T.);
#14257=ADVANCED_FACE('',(#1690),#1390,.T.);
#14258=ADVANCED_FACE('',(#1691),#1391,.T.);
#14259=ADVANCED_FACE('',(#1692),#581,.F.);
#14260=ADVANCED_FACE('',(#1693),#1392,.T.);
#14261=ADVANCED_FACE('',(#1694),#267,.T.);
#14262=ADVANCED_FACE('',(#1695),#1393,.T.);
#14263=ADVANCED_FACE('',(#1696),#582,.F.);
#14264=ADVANCED_FACE('',(#1697),#1394,.T.);
#14265=ADVANCED_FACE('',(#1698),#268,.T.);
#14266=ADVANCED_FACE('',(#1699),#1395,.T.);
#14267=ADVANCED_FACE('',(#1700),#583,.F.);
#14268=ADVANCED_FACE('',(#1701),#1396,.T.);
#14269=ADVANCED_FACE('',(#1702),#269,.T.);
#14270=ADVANCED_FACE('',(#1703),#1397,.T.);
#14271=ADVANCED_FACE('',(#1704),#270,.T.);
#14272=ADVANCED_FACE('',(#1705),#1398,.T.);
#14273=ADVANCED_FACE('',(#1706),#271,.T.);
#14274=ADVANCED_FACE('',(#1707),#1399,.T.);
#14275=ADVANCED_FACE('',(#1708),#272,.T.);
#14276=ADVANCED_FACE('',(#1709),#1400,.T.);
#14277=ADVANCED_FACE('',(#1710),#1401,.T.);
#14278=ADVANCED_FACE('',(#1711),#273,.T.);
#14279=ADVANCED_FACE('',(#1712,#429,#430),#1402,.F.);
#14280=ADVANCED_FACE('',(#1713),#207,.F.);
#14281=ADVANCED_FACE('',(#1714),#208,.F.);
#14282=ADVANCED_FACE('',(#1715),#209,.F.);
#14283=ADVANCED_FACE('',(#1716),#210,.F.);
#14284=ADVANCED_FACE('',(#1717),#211,.F.);
#14285=ADVANCED_FACE('',(#1718),#212,.F.);
#14286=ADVANCED_FACE('',(#1719),#213,.F.);
#14287=ADVANCED_FACE('',(#1720),#214,.F.);
#14288=ADVANCED_FACE('',(#1721),#1403,.F.);
#14289=ADVANCED_FACE('',(#1722),#584,.T.);
#14290=ADVANCED_FACE('',(#1723),#585,.T.);
#14291=ADVANCED_FACE('',(#1724),#586,.T.);
#14292=ADVANCED_FACE('',(#1725),#587,.T.);
#14293=ADVANCED_FACE('',(#1726),#1404,.F.);
#14294=ADVANCED_FACE('',(#1727,#431),#588,.F.);
#14295=ADVANCED_FACE('',(#1728),#1405,.F.);
#14296=ADVANCED_FACE('',(#1729,#432),#589,.F.);
#14297=ADVANCED_FACE('',(#1730),#1406,.F.);
#14298=ADVANCED_FACE('',(#1731,#433),#590,.F.);
#14299=ADVANCED_FACE('',(#1732,#434),#591,.T.);
#14300=ADVANCED_FACE('',(#1733),#1407,.T.);
#14301=ADVANCED_FACE('',(#1734),#1408,.T.);
#14302=ADVANCED_FACE('',(#1735),#592,.T.);
#14303=ADVANCED_FACE('',(#1736),#593,.T.);
#15071=CLOSED_SHELL('',(#14184,#14185,#14186,#14187,#14188,#14189,#14190,
#14191,#14192,#14193,#14194,#14195,#14196,#14197,#14198,#14199,#14200,#14201,
#14202,#14203,#14204,#14205,#14206,#14207,#14208,#14209,#14210,#14211,#14212,
#14213,#14214,#14215,#14216,#14217,#14218,#14219,#14220,#14221,#14222,#14223,
#14224,#14225,#14226,#14227,#14228,#14229,#14230,#14231,#14232,#14233,#14234,
#14235,#14236,#14237,#14238,#14239,#14240,#14241,#14242,#14243,#14244,#14245,
#14246,#14247,#14248,#14249,#14250,#14251,#14252,#14253,#14254,#14255,#14256,
#14257,#14258,#14259,#14260,#14261,#14262,#14263,#14264,#14265,#14266,#14267,
#14268,#14269,#14270,#14271,#14272,#14273,#14274,#14275,#14276,#14277,#14278,
#14279,#14280,#14281,#14282,#14283,#14284,#14285,#14286,#14287,#14288,#14289,
#14290,#14291,#14292,#14293,#14294,#14295,#14296,#14297,#14298,#14299,#14300,
#14301,#14302,#14303));
#15253=AXIS2_PLACEMENT_3D('',#20891,#16777,#16778);
#15254=AXIS2_PLACEMENT_3D('',#20892,#16779,#16780);
#15255=AXIS2_PLACEMENT_3D('',#20894,#16781,#16782);
#15256=AXIS2_PLACEMENT_3D('',#20897,#16784,#16785);
#15257=AXIS2_PLACEMENT_3D('',#20898,#16786,#16787);
#15258=AXIS2_PLACEMENT_3D('',#20902,#16789,#16790);
#15259=AXIS2_PLACEMENT_3D('',#20914,#16791,#16792);
#15260=AXIS2_PLACEMENT_3D('',#20915,#16793,#16794);
#15261=AXIS2_PLACEMENT_3D('',#20917,#16795,#16796);
#15262=AXIS2_PLACEMENT_3D('',#20918,#16797,#16798);
#15263=AXIS2_PLACEMENT_3D('',#20920,#16799,#16800);
#15264=AXIS2_PLACEMENT_3D('',#20923,#16802,#16803);
#15265=AXIS2_PLACEMENT_3D('',#20924,#16804,#16805);
#15266=AXIS2_PLACEMENT_3D('',#20929,#16807,#16808);
#15267=AXIS2_PLACEMENT_3D('',#20933,#16810,#16811);
#15268=AXIS2_PLACEMENT_3D('',#20936,#16813,#16814);
#15269=AXIS2_PLACEMENT_3D('',#20937,#16815,#16816);
#15270=AXIS2_PLACEMENT_3D('',#20939,#16817,#16818);
#15271=AXIS2_PLACEMENT_3D('',#20941,#16820,#16821);
#15272=AXIS2_PLACEMENT_3D('',#20943,#16822,#16823);
#15273=AXIS2_PLACEMENT_3D('',#20946,#16825,#16826);
#15274=AXIS2_PLACEMENT_3D('',#20947,#16827,#16828);
#15275=AXIS2_PLACEMENT_3D('',#20949,#16829,#16830);
#15276=AXIS2_PLACEMENT_3D('',#20950,#16831,#16832);
#15277=AXIS2_PLACEMENT_3D('',#20954,#16834,#16835);
#15278=AXIS2_PLACEMENT_3D('',#20966,#16836,#16837);
#15279=AXIS2_PLACEMENT_3D('',#20967,#16838,#16839);
#15280=AXIS2_PLACEMENT_3D('',#20969,#16840,#16841);
#15281=AXIS2_PLACEMENT_3D('',#20972,#16843,#16844);
#15282=AXIS2_PLACEMENT_3D('',#20973,#16845,#16846);
#15283=AXIS2_PLACEMENT_3D('',#20978,#16848,#16849);
#15284=AXIS2_PLACEMENT_3D('',#20982,#16851,#16852);
#15285=AXIS2_PLACEMENT_3D('',#20985,#16854,#16855);
#15286=AXIS2_PLACEMENT_3D('',#20986,#16856,#16857);
#15287=AXIS2_PLACEMENT_3D('',#20988,#16858,#16859);
#15288=AXIS2_PLACEMENT_3D('',#20990,#16861,#16862);
#15289=AXIS2_PLACEMENT_3D('',#20993,#16864,#16865);
#15290=AXIS2_PLACEMENT_3D('',#20994,#16866,#16867);
#15291=AXIS2_PLACEMENT_3D('',#21004,#16869,#16870);
#15292=AXIS2_PLACEMENT_3D('',#21014,#16871,#16872);
#15293=AXIS2_PLACEMENT_3D('',#21016,#16873,#16874);
#15294=AXIS2_PLACEMENT_3D('',#21019,#16876,#16877);
#15295=AXIS2_PLACEMENT_3D('',#21020,#16878,#16879);
#15296=AXIS2_PLACEMENT_3D('',#21025,#16881,#16882);
#15297=AXIS2_PLACEMENT_3D('',#21029,#16884,#16885);
#15298=AXIS2_PLACEMENT_3D('',#21033,#16887,#16888);
#15299=AXIS2_PLACEMENT_3D('',#21036,#16890,#16891);
#15300=AXIS2_PLACEMENT_3D('',#21038,#16892,#16893);
#15301=AXIS2_PLACEMENT_3D('',#21040,#16894,#16895);
#15302=AXIS2_PLACEMENT_3D('',#21042,#16896,#16897);
#15303=AXIS2_PLACEMENT_3D('',#21044,#16898,#16899);
#15304=AXIS2_PLACEMENT_3D('',#21045,#16900,#16901);
#15305=AXIS2_PLACEMENT_3D('',#21048,#16903,#16904);
#15306=AXIS2_PLACEMENT_3D('',#21049,#16905,#16906);
#15307=AXIS2_PLACEMENT_3D('',#21052,#16908,#16909);
#15308=AXIS2_PLACEMENT_3D('',#21053,#16910,#16911);
#15309=AXIS2_PLACEMENT_3D('',#21056,#16913,#16914);
#15310=AXIS2_PLACEMENT_3D('',#21057,#16915,#16916);
#15311=AXIS2_PLACEMENT_3D('',#21060,#16918,#16919);
#15312=AXIS2_PLACEMENT_3D('',#21061,#16920,#16921);
#15313=AXIS2_PLACEMENT_3D('',#21064,#16923,#16924);
#15314=AXIS2_PLACEMENT_3D('',#21065,#16925,#16926);
#15315=AXIS2_PLACEMENT_3D('',#21068,#16928,#16929);
#15316=AXIS2_PLACEMENT_3D('',#21069,#16930,#16931);
#15317=AXIS2_PLACEMENT_3D('',#21072,#16933,#16934);
#15318=AXIS2_PLACEMENT_3D('',#21073,#16935,#16936);
#15319=AXIS2_PLACEMENT_3D('',#21084,#16937,#16938);
#15320=AXIS2_PLACEMENT_3D('',#21093,#16939,#16940);
#15321=AXIS2_PLACEMENT_3D('',#21097,#16942,#16943);
#15322=AXIS2_PLACEMENT_3D('',#21099,#16945,#16946);
#15323=AXIS2_PLACEMENT_3D('',#21115,#16953,#16954);
#15324=AXIS2_PLACEMENT_3D('',#21131,#16956,#16957);
#15325=AXIS2_PLACEMENT_3D('',#21133,#16959,#16960);
#15326=AXIS2_PLACEMENT_3D('',#21170,#16969,#16970);
#15327=AXIS2_PLACEMENT_3D('',#21172,#16971,#16972);
#15328=AXIS2_PLACEMENT_3D('',#21185,#16974,#16975);
#15329=AXIS2_PLACEMENT_3D('',#21188,#16976,#16977);
#15330=AXIS2_PLACEMENT_3D('',#21205,#16978,#16979);
#15331=AXIS2_PLACEMENT_3D('',#21209,#16981,#16982);
#15332=AXIS2_PLACEMENT_3D('',#21211,#16984,#16985);
#15333=AXIS2_PLACEMENT_3D('',#21224,#16987,#16988);
#15334=AXIS2_PLACEMENT_3D('',#21245,#16990,#16991);
#15335=AXIS2_PLACEMENT_3D('',#21254,#16992,#16993);
#15336=AXIS2_PLACEMENT_3D('',#21265,#16994,#16995);
#15337=AXIS2_PLACEMENT_3D('',#21274,#16996,#16997);
#15338=AXIS2_PLACEMENT_3D('',#21285,#16998,#16999);
#15339=AXIS2_PLACEMENT_3D('',#21294,#17000,#17001);
#15340=AXIS2_PLACEMENT_3D('',#21298,#17003,#17004);
#15341=AXIS2_PLACEMENT_3D('',#21300,#17006,#17007);
#15342=AXIS2_PLACEMENT_3D('',#21310,#17013,#17014);
#15343=AXIS2_PLACEMENT_3D('',#21326,#17016,#17017);
#15344=AXIS2_PLACEMENT_3D('',#21328,#17019,#17020);
#15345=AXIS2_PLACEMENT_3D('',#21365,#17029,#17030);
#15346=AXIS2_PLACEMENT_3D('',#21367,#17031,#17032);
#15347=AXIS2_PLACEMENT_3D('',#21380,#17034,#17035);
#15348=AXIS2_PLACEMENT_3D('',#21383,#17036,#17037);
#15349=AXIS2_PLACEMENT_3D('',#21396,#17038,#17039);
#15350=AXIS2_PLACEMENT_3D('',#21398,#17040,#17041);
#15351=AXIS2_PLACEMENT_3D('',#21400,#17043,#17044);
#15352=AXIS2_PLACEMENT_3D('',#21413,#17046,#17047);
#15353=AXIS2_PLACEMENT_3D('',#21434,#17049,#17050);
#15354=AXIS2_PLACEMENT_3D('',#21443,#17051,#17052);
#15355=AXIS2_PLACEMENT_3D('',#21454,#17053,#17054);
#15356=AXIS2_PLACEMENT_3D('',#21463,#17055,#17056);
#15357=AXIS2_PLACEMENT_3D('',#21465,#17057,#17058);
#15358=AXIS2_PLACEMENT_3D('',#21467,#17060,#17061);
#15359=AXIS2_PLACEMENT_3D('',#21470,#17062,#17063);
#15360=AXIS2_PLACEMENT_3D('',#21474,#17065,#17066);
#15361=AXIS2_PLACEMENT_3D('',#21478,#17068,#17069);
#15362=AXIS2_PLACEMENT_3D('',#21482,#17071,#17072);
#15363=AXIS2_PLACEMENT_3D('',#21485,#17074,#17075);
#15364=AXIS2_PLACEMENT_3D('',#21487,#17076,#17077);
#15365=AXIS2_PLACEMENT_3D('',#21488,#17078,#17079);
#15366=AXIS2_PLACEMENT_3D('',#21490,#17081,#17082);
#15367=AXIS2_PLACEMENT_3D('',#21519,#17083,#17084);
#15368=AXIS2_PLACEMENT_3D('',#21521,#17085,#17086);
#15369=AXIS2_PLACEMENT_3D('',#21523,#17088,#17089);
#15370=AXIS2_PLACEMENT_3D('',#21525,#17090,#17091);
#15371=AXIS2_PLACEMENT_3D('',#21526,#17092,#17093);
#15372=AXIS2_PLACEMENT_3D('',#21527,#17094,#17095);
#15373=AXIS2_PLACEMENT_3D('',#21543,#17097,#17098);
#15374=AXIS2_PLACEMENT_3D('',#21558,#17099,#17100);
#15375=AXIS2_PLACEMENT_3D('',#21560,#17101,#17102);
#15376=AXIS2_PLACEMENT_3D('',#21562,#17103,#17104);
#15377=AXIS2_PLACEMENT_3D('',#21563,#17105,#17106);
#15378=AXIS2_PLACEMENT_3D('',#21564,#17107,#17108);
#15379=AXIS2_PLACEMENT_3D('',#21566,#17110,#17111);
#15380=AXIS2_PLACEMENT_3D('',#21568,#17113,#17114);
#15381=AXIS2_PLACEMENT_3D('',#21572,#17116,#17117);
#15382=AXIS2_PLACEMENT_3D('',#21574,#17119,#17120);
#15383=AXIS2_PLACEMENT_3D('',#21576,#17122,#17123);
#15384=AXIS2_PLACEMENT_3D('',#21577,#17124,#17125);
#15385=AXIS2_PLACEMENT_3D('',#21578,#17126,#17127);
#15386=AXIS2_PLACEMENT_3D('',#21580,#17128,#17129);
#15387=AXIS2_PLACEMENT_3D('',#21582,#17131,#17132);
#15388=AXIS2_PLACEMENT_3D('',#21584,#17133,#17134);
#15389=AXIS2_PLACEMENT_3D('',#21585,#17135,#17136);
#15390=AXIS2_PLACEMENT_3D('',#21586,#17137,#17138);
#15391=AXIS2_PLACEMENT_3D('',#21588,#17140,#17141);
#15392=AXIS2_PLACEMENT_3D('',#21590,#17143,#17144);
#15393=AXIS2_PLACEMENT_3D('',#21592,#17146,#17147);
#15394=AXIS2_PLACEMENT_3D('',#21593,#17148,#17149);
#15395=AXIS2_PLACEMENT_3D('',#21594,#17150,#17151);
#15396=AXIS2_PLACEMENT_3D('',#21595,#17152,#17153);
#15397=AXIS2_PLACEMENT_3D('',#21596,#17154,#17155);
#15398=AXIS2_PLACEMENT_3D('',#21598,#17157,#17158);
#15399=AXIS2_PLACEMENT_3D('',#21599,#17159,#17160);
#15400=AXIS2_PLACEMENT_3D('',#21600,#17161,#17162);
#15401=AXIS2_PLACEMENT_3D('',#21601,#17163,#17164);
#15402=AXIS2_PLACEMENT_3D('',#21602,#17165,#17166);
#15403=AXIS2_PLACEMENT_3D('',#21604,#17167,#17168);
#15404=AXIS2_PLACEMENT_3D('',#21606,#17169,#17170);
#15405=AXIS2_PLACEMENT_3D('',#21607,#17171,#17172);
#15406=AXIS2_PLACEMENT_3D('',#21608,#17173,#17174);
#15407=AXIS2_PLACEMENT_3D('',#21610,#17176,#17177);
#15408=AXIS2_PLACEMENT_3D('',#21613,#17179,#17180);
#15409=AXIS2_PLACEMENT_3D('',#21614,#17181,#17182);
#15410=AXIS2_PLACEMENT_3D('',#21616,#17183,#17184);
#15411=AXIS2_PLACEMENT_3D('',#21617,#17185,#17186);
#15412=AXIS2_PLACEMENT_3D('',#21618,#17187,#17188);
#15413=AXIS2_PLACEMENT_3D('',#21619,#17189,#17190);
#15414=AXIS2_PLACEMENT_3D('',#21621,#17192,#17193);
#15415=AXIS2_PLACEMENT_3D('',#21622,#17194,#17195);
#15416=AXIS2_PLACEMENT_3D('',#21624,#17196,#17197);
#15417=AXIS2_PLACEMENT_3D('',#21626,#17198,#17199);
#15418=AXIS2_PLACEMENT_3D('',#21627,#17200,#17201);
#15419=AXIS2_PLACEMENT_3D('',#21628,#17202,#17203);
#15420=AXIS2_PLACEMENT_3D('',#21629,#17204,#17205);
#15421=AXIS2_PLACEMENT_3D('',#21631,#17207,#17208);
#15422=AXIS2_PLACEMENT_3D('',#21633,#17210,#17211);
#15423=AXIS2_PLACEMENT_3D('',#21634,#17212,#17213);
#15424=AXIS2_PLACEMENT_3D('',#21637,#17215,#17216);
#15425=AXIS2_PLACEMENT_3D('',#21638,#17217,#17218);
#15426=AXIS2_PLACEMENT_3D('',#21640,#17219,#17220);
#15427=AXIS2_PLACEMENT_3D('',#21641,#17221,#17222);
#15428=AXIS2_PLACEMENT_3D('',#21642,#17223,#17224);
#15429=AXIS2_PLACEMENT_3D('',#21643,#17225,#17226);
#15430=AXIS2_PLACEMENT_3D('',#21645,#17228,#17229);
#15431=AXIS2_PLACEMENT_3D('',#21646,#17230,#17231);
#15432=AXIS2_PLACEMENT_3D('',#21649,#17233,#17234);
#15433=AXIS2_PLACEMENT_3D('',#21650,#17235,#17236);
#15434=AXIS2_PLACEMENT_3D('',#21652,#17237,#17238);
#15435=AXIS2_PLACEMENT_3D('',#21653,#17239,#17240);
#15436=AXIS2_PLACEMENT_3D('',#21654,#17241,#17242);
#15437=AXIS2_PLACEMENT_3D('',#21655,#17243,#17244);
#15438=AXIS2_PLACEMENT_3D('',#21657,#17246,#17247);
#15439=AXIS2_PLACEMENT_3D('',#21658,#17248,#17249);
#15440=AXIS2_PLACEMENT_3D('',#21659,#17250,#17251);
#15441=AXIS2_PLACEMENT_3D('',#21660,#17252,#17253);
#15442=AXIS2_PLACEMENT_3D('',#21661,#17254,#17255);
#15443=AXIS2_PLACEMENT_3D('',#21662,#17256,#17257);
#15444=AXIS2_PLACEMENT_3D('',#21663,#17258,#17259);
#15445=AXIS2_PLACEMENT_3D('',#21664,#17260,#17261);
#15446=AXIS2_PLACEMENT_3D('',#21665,#17262,#17263);
#15447=AXIS2_PLACEMENT_3D('',#21666,#17264,#17265);
#15448=AXIS2_PLACEMENT_3D('',#21667,#17266,#17267);
#15449=AXIS2_PLACEMENT_3D('',#21668,#17268,#17269);
#15450=AXIS2_PLACEMENT_3D('',#21669,#17270,#17271);
#15451=AXIS2_PLACEMENT_3D('',#21670,#17272,#17273);
#15452=AXIS2_PLACEMENT_3D('',#21671,#17274,#17275);
#15453=AXIS2_PLACEMENT_3D('',#21672,#17276,#17277);
#15454=AXIS2_PLACEMENT_3D('',#21673,#17278,#17279);
#15455=AXIS2_PLACEMENT_3D('',#21674,#17280,#17281);
#15456=AXIS2_PLACEMENT_3D('',#21675,#17282,#17283);
#15457=AXIS2_PLACEMENT_3D('',#21676,#17284,#17285);
#15458=AXIS2_PLACEMENT_3D('',#21677,#17286,#17287);
#15459=AXIS2_PLACEMENT_3D('',#21678,#17288,#17289);
#15460=AXIS2_PLACEMENT_3D('',#21679,#17290,#17291);
#15461=AXIS2_PLACEMENT_3D('',#21680,#17292,#17293);
#15462=AXIS2_PLACEMENT_3D('',#21682,#17294,#17295);
#15463=AXIS2_PLACEMENT_3D('',#21684,#17296,#17297);
#15464=AXIS2_PLACEMENT_3D('',#21685,#17298,#17299);
#15465=AXIS2_PLACEMENT_3D('',#21686,#17300,#17301);
#15466=AXIS2_PLACEMENT_3D('',#21688,#17302,#17303);
#15467=AXIS2_PLACEMENT_3D('',#22095,#17305,#17306);
#15468=AXIS2_PLACEMENT_3D('',#22178,#17307,#17308);
#15469=AXIS2_PLACEMENT_3D('',#22399,#17309,#17310);
#15470=AXIS2_PLACEMENT_3D('',#22483,#17311,#17312);
#15471=AXIS2_PLACEMENT_3D('',#22484,#17313,#17314);
#15472=AXIS2_PLACEMENT_3D('',#22594,#17315,#17316);
#15473=AXIS2_PLACEMENT_3D('',#22596,#17318,#17319);
#15474=AXIS2_PLACEMENT_3D('',#22597,#17320,#17321);
#15475=AXIS2_PLACEMENT_3D('',#22598,#17322,#17323);
#15476=AXIS2_PLACEMENT_3D('',#22599,#17324,#17325);
#15477=AXIS2_PLACEMENT_3D('',#22600,#17326,#17327);
#15478=AXIS2_PLACEMENT_3D('',#22602,#17328,#17329);
#15479=AXIS2_PLACEMENT_3D('',#22605,#17331,#17332);
#15480=AXIS2_PLACEMENT_3D('',#22606,#17333,#17334);
#15481=AXIS2_PLACEMENT_3D('',#22608,#17335,#17336);
#15482=AXIS2_PLACEMENT_3D('',#22609,#17337,#17338);
#15483=AXIS2_PLACEMENT_3D('',#22612,#17340,#17341);
#15484=AXIS2_PLACEMENT_3D('',#22613,#17342,#17343);
#15485=AXIS2_PLACEMENT_3D('',#22615,#17344,#17345);
#15486=AXIS2_PLACEMENT_3D('',#22616,#17346,#17347);
#15487=AXIS2_PLACEMENT_3D('',#22619,#17349,#17350);
#15488=AXIS2_PLACEMENT_3D('',#22620,#17351,#17352);
#15489=AXIS2_PLACEMENT_3D('',#22621,#17353,#17354);
#15490=AXIS2_PLACEMENT_3D('',#22622,#17355,#17356);
#15491=AXIS2_PLACEMENT_3D('',#22623,#17357,#17358);
#15492=AXIS2_PLACEMENT_3D('',#22624,#17359,#17360);
#15493=AXIS2_PLACEMENT_3D('',#22625,#17361,#17362);
#16777=DIRECTION('axis',(0.,0.,1.));
#16778=DIRECTION('refdir',(1.,0.,0.));
#16779=DIRECTION('center_axis',(0.,0.,1.));
#16780=DIRECTION('ref_axis',(1.,0.,0.));
#16781=DIRECTION('center_axis',(0.,0.,1.));
#16782=DIRECTION('ref_axis',(1.,0.,0.));
#16783=DIRECTION('',(-0.707106781186548,8.65956056235493E-17,0.707106781186548));
#16784=DIRECTION('center_axis',(0.,0.,-1.));
#16785=DIRECTION('ref_axis',(1.,0.,0.));
#16786=DIRECTION('center_axis',(0.,0.,-1.));
#16787=DIRECTION('ref_axis',(1.,0.,0.));
#16788=DIRECTION('',(0.,0.,1.));
#16789=DIRECTION('center_axis',(0.,0.,1.));
#16790=DIRECTION('ref_axis',(1.,0.,0.));
#16791=DIRECTION('center_axis',(0.,0.,1.));
#16792=DIRECTION('ref_axis',(1.,0.,0.));
#16793=DIRECTION('center_axis',(0.,0.,1.));
#16794=DIRECTION('ref_axis',(1.,0.,0.));
#16795=DIRECTION('center_axis',(0.,0.,1.));
#16796=DIRECTION('ref_axis',(1.,0.,0.));
#16797=DIRECTION('center_axis',(1.,0.,0.));
#16798=DIRECTION('ref_axis',(0.,0.,-1.));
#16799=DIRECTION('center_axis',(1.,0.,0.));
#16800=DIRECTION('ref_axis',(0.,0.,-1.));
#16801=DIRECTION('',(-0.707106781186548,8.65956056235493E-17,-0.707106781186548));
#16802=DIRECTION('center_axis',(-1.,0.,0.));
#16803=DIRECTION('ref_axis',(0.,0.,-1.));
#16804=DIRECTION('center_axis',(1.,0.,0.));
#16805=DIRECTION('ref_axis',(0.,0.,-1.));
#16806=DIRECTION('',(0.,-1.,0.));
#16807=DIRECTION('center_axis',(-1.,0.,0.));
#16808=DIRECTION('ref_axis',(0.,0.,-1.));
#16809=DIRECTION('',(0.,0.,1.));
#16810=DIRECTION('center_axis',(-1.,0.,0.));
#16811=DIRECTION('ref_axis',(0.,0.,1.));
#16812=DIRECTION('',(0.,1.,0.));
#16813=DIRECTION('center_axis',(-1.,0.,0.));
#16814=DIRECTION('ref_axis',(0.,-1.,1.83697019872103E-16));
#16815=DIRECTION('center_axis',(1.,0.,0.));
#16816=DIRECTION('ref_axis',(0.,0.,-1.));
#16817=DIRECTION('center_axis',(1.,0.,0.));
#16818=DIRECTION('ref_axis',(0.,0.,-1.));
#16819=DIRECTION('',(1.,0.,0.));
#16820=DIRECTION('center_axis',(0.,0.,-1.));
#16821=DIRECTION('ref_axis',(1.,0.,0.));
#16822=DIRECTION('center_axis',(0.,0.,-1.));
#16823=DIRECTION('ref_axis',(1.,0.,0.));
#16824=DIRECTION('',(-0.707106781186548,-8.65956056235493E-17,-0.707106781186548));
#16825=DIRECTION('center_axis',(0.,0.,1.));
#16826=DIRECTION('ref_axis',(1.,0.,0.));
#16827=DIRECTION('center_axis',(0.,0.,1.));
#16828=DIRECTION('ref_axis',(1.,0.,0.));
#16829=DIRECTION('center_axis',(0.,0.,1.));
#16830=DIRECTION('ref_axis',(1.,0.,0.));
#16831=DIRECTION('center_axis',(0.,0.,1.));
#16832=DIRECTION('ref_axis',(1.,0.,0.));
#16833=DIRECTION('',(0.,0.,-1.));
#16834=DIRECTION('center_axis',(0.,0.,-1.));
#16835=DIRECTION('ref_axis',(1.,0.,0.));
#16836=DIRECTION('center_axis',(0.,0.,-1.));
#16837=DIRECTION('ref_axis',(1.,0.,0.));
#16838=DIRECTION('center_axis',(1.,0.,0.));
#16839=DIRECTION('ref_axis',(0.,0.,-1.));
#16840=DIRECTION('center_axis',(1.,0.,0.));
#16841=DIRECTION('ref_axis',(0.,0.,-1.));
#16842=DIRECTION('',(-0.707106781186548,8.65956056235493E-17,-0.707106781186548));
#16843=DIRECTION('center_axis',(-1.,0.,0.));
#16844=DIRECTION('ref_axis',(0.,0.,-1.));
#16845=DIRECTION('center_axis',(1.,0.,0.));
#16846=DIRECTION('ref_axis',(0.,0.,-1.));
#16847=DIRECTION('',(0.,-1.,0.));
#16848=DIRECTION('center_axis',(-1.,0.,0.));
#16849=DIRECTION('ref_axis',(0.,1.,-6.12323399573677E-17));
#16850=DIRECTION('',(0.,1.,0.));
#16851=DIRECTION('center_axis',(-1.,0.,0.));
#16852=DIRECTION('ref_axis',(0.,0.,1.));
#16853=DIRECTION('',(0.,0.,-1.));
#16854=DIRECTION('center_axis',(-1.,0.,0.));
#16855=DIRECTION('ref_axis',(0.,0.,-1.));
#16856=DIRECTION('center_axis',(1.,0.,0.));
#16857=DIRECTION('ref_axis',(0.,0.,-1.));
#16858=DIRECTION('center_axis',(1.,0.,0.));
#16859=DIRECTION('ref_axis',(0.,0.,-1.));
#16860=DIRECTION('',(1.,0.,0.));
#16861=DIRECTION('center_axis',(0.,0.,1.));
#16862=DIRECTION('ref_axis',(1.,0.,0.));
#16863=DIRECTION('',(0.707106781186547,8.65956056235493E-17,-0.707106781186547));
#16864=DIRECTION('center_axis',(0.,0.,-1.));
#16865=DIRECTION('ref_axis',(1.,0.,0.));
#16866=DIRECTION('center_axis',(0.,0.,-1.));
#16867=DIRECTION('ref_axis',(1.,0.,0.));
#16868=DIRECTION('',(0.,0.,-1.));
#16869=DIRECTION('center_axis',(0.,0.,-1.));
#16870=DIRECTION('ref_axis',(1.,0.,0.));
#16871=DIRECTION('center_axis',(1.,0.,0.));
#16872=DIRECTION('ref_axis',(0.,0.,-1.));
#16873=DIRECTION('center_axis',(1.,0.,0.));
#16874=DIRECTION('ref_axis',(0.,0.,-1.));
#16875=DIRECTION('',(-0.707106781186554,8.65956056235486E-17,-0.707106781186541));
#16876=DIRECTION('center_axis',(-1.,0.,0.));
#16877=DIRECTION('ref_axis',(0.,0.,-1.));
#16878=DIRECTION('center_axis',(1.,0.,0.));
#16879=DIRECTION('ref_axis',(0.,0.,-1.));
#16880=DIRECTION('',(0.,-1.,0.));
#16881=DIRECTION('center_axis',(-1.,0.,0.));
#16882=DIRECTION('ref_axis',(0.,0.707106781186547,-0.707106781186547));
#16883=DIRECTION('',(0.,0.,-1.));
#16884=DIRECTION('center_axis',(-1.,0.,0.));
#16885=DIRECTION('ref_axis',(0.,0.707106781186547,0.707106781186547));
#16886=DIRECTION('',(0.,1.,0.));
#16887=DIRECTION('center_axis',(-1.,0.,0.));
#16888=DIRECTION('ref_axis',(0.,-0.707106781186547,0.707106781186547));
#16889=DIRECTION('',(0.,0.,1.));
#16890=DIRECTION('center_axis',(-1.,0.,0.));
#16891=DIRECTION('ref_axis',(0.,-0.707106781186547,-0.707106781186547));
#16892=DIRECTION('center_axis',(1.,0.,0.));
#16893=DIRECTION('ref_axis',(0.,0.,-1.));
#16894=DIRECTION('center_axis',(1.,0.,0.));
#16895=DIRECTION('ref_axis',(0.,0.,-1.));
#16896=DIRECTION('center_axis',(1.,0.,0.));
#16897=DIRECTION('ref_axis',(0.,1.,0.));
#16898=DIRECTION('center_axis',(1.,0.,0.));
#16899=DIRECTION('ref_axis',(0.,0.,-1.));
#16900=DIRECTION('center_axis',(-1.,0.,0.));
#16901=DIRECTION('ref_axis',(0.,0.,-1.));
#16902=DIRECTION('',(-1.,0.,0.));
#16903=DIRECTION('center_axis',(-1.,0.,0.));
#16904=DIRECTION('ref_axis',(0.,0.,-1.));
#16905=DIRECTION('center_axis',(1.,0.,0.));
#16906=DIRECTION('ref_axis',(0.,0.,-1.));
#16907=DIRECTION('',(-0.707106781186554,8.65956056235486E-17,-0.707106781186541));
#16908=DIRECTION('center_axis',(-1.,0.,0.));
#16909=DIRECTION('ref_axis',(0.,0.,-1.));
#16910=DIRECTION('center_axis',(-1.,0.,0.));
#16911=DIRECTION('ref_axis',(0.,0.,-1.));
#16912=DIRECTION('',(-1.,0.,0.));
#16913=DIRECTION('center_axis',(-1.,0.,0.));
#16914=DIRECTION('ref_axis',(0.,0.,-1.));
#16915=DIRECTION('center_axis',(1.,0.,0.));
#16916=DIRECTION('ref_axis',(0.,0.,-1.));
#16917=DIRECTION('',(-0.707106781186554,8.65956056235486E-17,-0.707106781186541));
#16918=DIRECTION('center_axis',(-1.,0.,0.));
#16919=DIRECTION('ref_axis',(0.,0.,-1.));
#16920=DIRECTION('center_axis',(-1.,0.,0.));
#16921=DIRECTION('ref_axis',(0.,0.,-1.));
#16922=DIRECTION('',(-1.,0.,0.));
#16923=DIRECTION('center_axis',(-1.,0.,0.));
#16924=DIRECTION('ref_axis',(0.,0.,-1.));
#16925=DIRECTION('center_axis',(1.,0.,0.));
#16926=DIRECTION('ref_axis',(0.,0.,-1.));
#16927=DIRECTION('',(-0.707106781186554,8.65956056235486E-17,-0.707106781186541));
#16928=DIRECTION('center_axis',(-1.,0.,0.));
#16929=DIRECTION('ref_axis',(0.,0.,-1.));
#16930=DIRECTION('center_axis',(-1.,0.,0.));
#16931=DIRECTION('ref_axis',(0.,0.,-1.));
#16932=DIRECTION('',(-1.,0.,0.));
#16933=DIRECTION('center_axis',(-1.,0.,0.));
#16934=DIRECTION('ref_axis',(0.,0.,-1.));
#16935=DIRECTION('center_axis',(-1.,0.,0.));
#16936=DIRECTION('ref_axis',(0.,0.,-1.));
#16937=DIRECTION('center_axis',(1.,0.,0.));
#16938=DIRECTION('ref_axis',(0.,0.,-1.));
#16939=DIRECTION('center_axis',(0.,-0.989664670474115,-0.143400976340336));
#16940=DIRECTION('ref_axis',(0.,0.143400976340336,-0.989664670474115));
#16941=DIRECTION('',(1.,0.,0.));
#16942=DIRECTION('center_axis',(0.,-0.989664670474115,-0.143400976340336));
#16943=DIRECTION('ref_axis',(0.,-0.143400976340336,0.989664670474115));
#16944=DIRECTION('',(-1.,0.,0.));
#16945=DIRECTION('center_axis',(0.,-1.,0.));
#16946=DIRECTION('ref_axis',(0.,0.,-1.));
#16947=DIRECTION('',(0.,0.,1.));
#16948=DIRECTION('',(1.,0.,0.));
#16949=DIRECTION('',(0.,0.,-1.));
#16950=DIRECTION('',(1.,0.,0.));
#16951=DIRECTION('',(0.,0.,1.));
#16952=DIRECTION('',(1.,0.,0.));
#16953=DIRECTION('center_axis',(0.,-0.143400976340336,-0.989664670474115));
#16954=DIRECTION('ref_axis',(-1.,0.,0.));
#16955=DIRECTION('',(1.,0.,0.));
#16956=DIRECTION('center_axis',(0.,-0.143400976340336,-0.989664670474115));
#16957=DIRECTION('ref_axis',(0.,0.989664670474115,-0.143400976340336));
#16958=DIRECTION('',(-1.,0.,0.));
#16959=DIRECTION('center_axis',(0.,0.,-1.));
#16960=DIRECTION('ref_axis',(0.,1.,0.));
#16961=DIRECTION('',(0.,-1.,0.));
#16962=DIRECTION('',(0.,-1.,0.));
#16963=DIRECTION('',(-1.,0.,0.));
#16964=DIRECTION('',(0.,-1.,0.));
#16965=DIRECTION('',(1.,0.,0.));
#16966=DIRECTION('',(1.,0.,0.));
#16967=DIRECTION('',(0.,1.,0.));
#16968=DIRECTION('',(1.,0.,0.));
#16969=DIRECTION('center_axis',(0.,0.143400976340336,-0.989664670474115));
#16970=DIRECTION('ref_axis',(-1.,0.,0.));
#16971=DIRECTION('center_axis',(0.,0.143400976340336,-0.989664670474115));
#16972=DIRECTION('ref_axis',(0.,-0.989664670474115,-0.143400976340336));
#16973=DIRECTION('',(1.,0.,0.));
#16974=DIRECTION('center_axis',(-1.,0.,0.));
#16975=DIRECTION('ref_axis',(0.,0.,-1.));
#16976=DIRECTION('center_axis',(1.,0.,0.));
#16977=DIRECTION('ref_axis',(0.,0.,-1.));
#16978=DIRECTION('center_axis',(0.,0.989664670474115,-0.143400976340336));
#16979=DIRECTION('ref_axis',(0.,0.143400976340336,0.989664670474115));
#16980=DIRECTION('',(1.,0.,0.));
#16981=DIRECTION('center_axis',(0.,0.989664670474115,-0.143400976340336));
#16982=DIRECTION('ref_axis',(0.,0.143400976340336,0.989664670474115));
#16983=DIRECTION('',(-1.,0.,0.));
#16984=DIRECTION('center_axis',(1.,0.,0.));
#16985=DIRECTION('ref_axis',(0.,0.,-1.));
#16986=DIRECTION('',(1.,0.,0.));
#16987=DIRECTION('center_axis',(-1.,0.,0.));
#16988=DIRECTION('ref_axis',(0.,-1.11022302462516E-16,-1.));
#16989=DIRECTION('',(1.,0.,0.));
#16990=DIRECTION('center_axis',(1.,0.,0.));
#16991=DIRECTION('ref_axis',(0.,0.,-1.));
#16992=DIRECTION('center_axis',(1.,0.,0.));
#16993=DIRECTION('ref_axis',(0.,0.,-1.));
#16994=DIRECTION('center_axis',(1.,0.,0.));
#16995=DIRECTION('ref_axis',(0.,0.,-1.));
#16996=DIRECTION('center_axis',(-1.,0.,0.));
#16997=DIRECTION('ref_axis',(0.,0.,1.));
#16998=DIRECTION('center_axis',(1.,0.,0.));
#16999=DIRECTION('ref_axis',(0.,0.,1.));
#17000=DIRECTION('center_axis',(0.,0.989664670474115,0.143400976340336));
#17001=DIRECTION('ref_axis',(0.,-0.143400976340336,0.989664670474115));
#17002=DIRECTION('',(1.,0.,0.));
#17003=DIRECTION('center_axis',(0.,0.989664670474115,0.143400976340336));
#17004=DIRECTION('ref_axis',(0.,0.143400976340336,-0.989664670474115));
#17005=DIRECTION('',(-1.,0.,0.));
#17006=DIRECTION('center_axis',(0.,1.,0.));
#17007=DIRECTION('ref_axis',(0.,0.,1.));
#17008=DIRECTION('',(0.,0.,-1.));
#17009=DIRECTION('',(1.,0.,0.));
#17010=DIRECTION('',(0.,0.,1.));
#17011=DIRECTION('',(1.,0.,0.));
#17012=DIRECTION('',(0.,0.,-1.));
#17013=DIRECTION('center_axis',(0.,0.143400976340336,0.989664670474115));
#17014=DIRECTION('ref_axis',(1.,0.,0.));
#17015=DIRECTION('',(1.,0.,0.));
#17016=DIRECTION('center_axis',(0.,0.143400976340336,0.989664670474115));
#17017=DIRECTION('ref_axis',(0.,-0.989664670474115,0.143400976340336));
#17018=DIRECTION('',(-1.,0.,0.));
#17019=DIRECTION('center_axis',(0.,0.,1.));
#17020=DIRECTION('ref_axis',(0.,-1.,0.));
#17021=DIRECTION('',(0.,1.,0.));
#17022=DIRECTION('',(0.,1.,0.));
#17023=DIRECTION('',(-1.,0.,0.));
#17024=DIRECTION('',(0.,1.,0.));
#17025=DIRECTION('',(1.,0.,0.));
#17026=DIRECTION('',(0.,-1.,0.));
#17027=DIRECTION('',(1.,0.,0.));
#17028=DIRECTION('',(1.,0.,0.));
#17029=DIRECTION('center_axis',(0.,-0.143400976340336,0.989664670474115));
#17030=DIRECTION('ref_axis',(1.,0.,0.));
#17031=DIRECTION('center_axis',(0.,-0.143400976340336,0.989664670474115));
#17032=DIRECTION('ref_axis',(0.,0.989664670474115,0.143400976340336));
#17033=DIRECTION('',(1.,0.,0.));
#17034=DIRECTION('center_axis',(-1.,0.,0.));
#17035=DIRECTION('ref_axis',(0.,0.,1.));
#17036=DIRECTION('center_axis',(1.,0.,0.));
#17037=DIRECTION('ref_axis',(0.,0.,1.));
#17038=DIRECTION('center_axis',(0.,-0.989664670474115,0.143400976340336));
#17039=DIRECTION('ref_axis',(0.,-0.143400976340336,-0.989664670474115));
#17040=DIRECTION('center_axis',(0.,-0.989664670474115,0.143400976340336));
#17041=DIRECTION('ref_axis',(0.,-0.143400976340336,-0.989664670474115));
#17042=DIRECTION('',(-1.,0.,0.));
#17043=DIRECTION('center_axis',(1.,0.,0.));
#17044=DIRECTION('ref_axis',(0.,1.22464679914735E-16,1.));
#17045=DIRECTION('',(1.,0.,0.));
#17046=DIRECTION('center_axis',(-1.,0.,0.));
#17047=DIRECTION('ref_axis',(0.,0.0163578624861081,0.999866201216386));
#17048=DIRECTION('',(1.,0.,0.));
#17049=DIRECTION('center_axis',(1.,0.,0.));
#17050=DIRECTION('ref_axis',(0.,0.,-1.));
#17051=DIRECTION('center_axis',(1.,0.,0.));
#17052=DIRECTION('ref_axis',(0.,1.22464679914735E-16,1.));
#17053=DIRECTION('center_axis',(1.,0.,0.));
#17054=DIRECTION('ref_axis',(0.,0.,-1.));
#17055=DIRECTION('center_axis',(-1.,0.,0.));
#17056=DIRECTION('ref_axis',(0.,0.,-1.));
#17057=DIRECTION('center_axis',(-1.,0.,0.));
#17058=DIRECTION('ref_axis',(0.,0.,-1.));
#17059=DIRECTION('',(0.707106781186547,-8.65956056235494E-17,-0.707106781186548));
#17060=DIRECTION('center_axis',(1.,0.,0.));
#17061=DIRECTION('ref_axis',(0.,0.,-1.));
#17062=DIRECTION('center_axis',(1.,0.,0.));
#17063=DIRECTION('ref_axis',(0.,-1.11022302462516E-16,-1.));
#17064=DIRECTION('',(0.,1.,0.));
#17065=DIRECTION('center_axis',(1.,0.,0.));
#17066=DIRECTION('ref_axis',(0.,-1.,1.83697019872103E-16));
#17067=DIRECTION('',(0.,-1.,0.));
#17068=DIRECTION('center_axis',(1.,0.,0.));
#17069=DIRECTION('ref_axis',(0.,0.0163578624861081,0.999866201216386));
#17070=DIRECTION('',(0.,-1.,0.));
#17071=DIRECTION('center_axis',(1.,0.,0.));
#17072=DIRECTION('ref_axis',(0.,1.,-6.12323399573677E-17));
#17073=DIRECTION('',(0.,1.,0.));
#17074=DIRECTION('center_axis',(-1.,0.,0.));
#17075=DIRECTION('ref_axis',(0.,0.,-1.));
#17076=DIRECTION('center_axis',(1.,0.,0.));
#17077=DIRECTION('ref_axis',(0.,1.,0.));
#17078=DIRECTION('center_axis',(-1.,0.,0.));
#17079=DIRECTION('ref_axis',(0.,0.,-1.));
#17080=DIRECTION('',(0.707106781186547,-8.65956056235494E-17,-0.707106781186548));
#17081=DIRECTION('center_axis',(1.,0.,0.));
#17082=DIRECTION('ref_axis',(0.,-1.22464679914735E-16,1.));
#17083=DIRECTION('center_axis',(0.,-1.,0.));
#17084=DIRECTION('ref_axis',(-0.707106781186548,0.,0.707106781186547));
#17085=DIRECTION('center_axis',(0.,1.,-4.44089209850063E-15));
#17086=DIRECTION('ref_axis',(-1.,0.,0.));
#17087=DIRECTION('',(0.,1.,0.));
#17088=DIRECTION('center_axis',(1.,0.,0.));
#17089=DIRECTION('ref_axis',(0.,0.,-1.));
#17090=DIRECTION('center_axis',(0.,-1.,0.));
#17091=DIRECTION('ref_axis',(-1.,0.,0.));
#17092=DIRECTION('center_axis',(-1.,0.,0.));
#17093=DIRECTION('ref_axis',(0.,-1.,1.83697019872103E-16));
#17094=DIRECTION('center_axis',(0.,1.,0.));
#17095=DIRECTION('ref_axis',(-0.707106781186548,0.,-0.707106781186547));
#17096=DIRECTION('',(0.,-1.,0.));
#17097=DIRECTION('center_axis',(1.,0.,0.));
#17098=DIRECTION('ref_axis',(0.,0.,-1.));
#17099=DIRECTION('center_axis',(1.,0.,0.));
#17100=DIRECTION('ref_axis',(0.,0.,-1.));
#17101=DIRECTION('center_axis',(0.,1.,0.));
#17102=DIRECTION('ref_axis',(0.,0.,-1.));
#17103=DIRECTION('center_axis',(0.,1.,0.));
#17104=DIRECTION('ref_axis',(-1.,0.,0.));
#17105=DIRECTION('center_axis',(-1.,0.,0.));
#17106=DIRECTION('ref_axis',(0.,1.,-6.12323399573677E-17));
#17107=DIRECTION('center_axis',(0.,-1.,0.));
#17108=DIRECTION('ref_axis',(-0.707106781186548,0.,0.707106781186547));
#17109=DIRECTION('',(0.,1.,0.));
#17110=DIRECTION('center_axis',(0.,1.,0.));
#17111=DIRECTION('ref_axis',(-0.707106781186548,0.,-0.707106781186547));
#17112=DIRECTION('',(0.,-1.,0.));
#17113=DIRECTION('center_axis',(1.,0.,0.));
#17114=DIRECTION('ref_axis',(0.,0.,-1.));
#17115=DIRECTION('',(1.,0.,0.));
#17116=DIRECTION('center_axis',(1.,0.,0.));
#17117=DIRECTION('ref_axis',(0.,1.,-6.12323399573677E-17));
#17118=DIRECTION('',(1.,0.,0.));
#17119=DIRECTION('center_axis',(0.,0.,1.));
#17120=DIRECTION('ref_axis',(0.,-1.,0.));
#17121=DIRECTION('',(0.,-1.,0.));
#17122=DIRECTION('center_axis',(1.,0.,0.));
#17123=DIRECTION('ref_axis',(0.,1.22464679914735E-16,1.));
#17124=DIRECTION('center_axis',(-1.,0.,0.));
#17125=DIRECTION('ref_axis',(0.,1.22464679914735E-16,1.));
#17126=DIRECTION('center_axis',(0.,-1.,0.));
#17127=DIRECTION('ref_axis',(0.707106781186548,0.,0.707106781186548));
#17128=DIRECTION('center_axis',(0.,1.,-4.44089209850063E-15));
#17129=DIRECTION('ref_axis',(0.,4.44089209850063E-15,1.));
#17130=DIRECTION('',(0.,-1.,0.));
#17131=DIRECTION('center_axis',(1.,0.,0.));
#17132=DIRECTION('ref_axis',(0.,0.,-1.));
#17133=DIRECTION('center_axis',(0.,-1.,0.));
#17134=DIRECTION('ref_axis',(0.,0.,-1.));
#17135=DIRECTION('center_axis',(1.,0.,0.));
#17136=DIRECTION('ref_axis',(0.,-1.,1.83697019872103E-16));
#17137=DIRECTION('center_axis',(0.,1.,0.));
#17138=DIRECTION('ref_axis',(0.707106781186548,0.,-0.707106781186548));
#17139=DIRECTION('',(0.,1.,0.));
#17140=DIRECTION('center_axis',(0.,0.,-1.));
#17141=DIRECTION('ref_axis',(0.,1.,0.));
#17142=DIRECTION('',(1.,0.,0.));
#17143=DIRECTION('center_axis',(1.,0.,0.));
#17144=DIRECTION('ref_axis',(0.,0.,-1.));
#17145=DIRECTION('',(1.,0.,0.));
#17146=DIRECTION('center_axis',(0.,0.,1.));
#17147=DIRECTION('ref_axis',(0.,-1.,0.));
#17148=DIRECTION('center_axis',(1.,0.,0.));
#17149=DIRECTION('ref_axis',(0.,0.,-1.));
#17150=DIRECTION('center_axis',(-1.,0.,0.));
#17151=DIRECTION('ref_axis',(0.,0.,-1.));
#17152=DIRECTION('center_axis',(0.,1.,0.));
#17153=DIRECTION('ref_axis',(0.707106781186548,0.,-0.707106781186548));
#17154=DIRECTION('center_axis',(0.,-1.,4.44089209850063E-15));
#17155=DIRECTION('ref_axis',(0.,-4.44089209850063E-15,-1.));
#17156=DIRECTION('',(0.,1.,0.));
#17157=DIRECTION('center_axis',(1.,0.,0.));
#17158=DIRECTION('ref_axis',(0.,0.,-1.));
#17159=DIRECTION('center_axis',(0.,1.,0.));
#17160=DIRECTION('ref_axis',(0.,0.,1.));
#17161=DIRECTION('center_axis',(0.,-1.,0.));
#17162=DIRECTION('ref_axis',(0.707106781186548,0.,0.707106781186548));
#17163=DIRECTION('center_axis',(0.,0.,-1.));
#17164=DIRECTION('ref_axis',(0.,1.,0.));
#17165=DIRECTION('center_axis',(1.,0.,0.));
#17166=DIRECTION('ref_axis',(0.,1.,-1.84400444715477E-16));
#17167=DIRECTION('center_axis',(-1.,0.,0.));
#17168=DIRECTION('ref_axis',(0.,1.,-1.84400444715477E-16));
#17169=DIRECTION('center_axis',(0.,-3.06865124630212E-16,-1.));
#17170=DIRECTION('ref_axis',(0.,-1.,3.06865124630213E-16));
#17171=DIRECTION('center_axis',(1.,0.,0.));
#17172=DIRECTION('ref_axis',(0.,0.,-1.));
#17173=DIRECTION('center_axis',(1.,0.,0.));
#17174=DIRECTION('ref_axis',(0.,1.,0.));
#17175=DIRECTION('',(-1.,0.,0.));
#17176=DIRECTION('center_axis',(0.,-1.,0.));
#17177=DIRECTION('ref_axis',(-0.707106781186545,0.,0.70710678118655));
#17178=DIRECTION('',(0.,-1.,0.));
#17179=DIRECTION('center_axis',(0.,1.,-2.22044604925031E-15));
#17180=DIRECTION('ref_axis',(-1.,0.,0.));
#17181=DIRECTION('center_axis',(1.,0.,0.));
#17182=DIRECTION('ref_axis',(0.,0.,-1.));
#17183=DIRECTION('center_axis',(0.,0.,1.));
#17184=DIRECTION('ref_axis',(-1.,0.,0.));
#17185=DIRECTION('center_axis',(-1.,0.,0.));
#17186=DIRECTION('ref_axis',(0.,-0.707106781186548,0.707106781186548));
#17187=DIRECTION('center_axis',(1.,0.,0.));
#17188=DIRECTION('ref_axis',(0.,-0.707106781186547,0.707106781186547));
#17189=DIRECTION('center_axis',(0.,0.,-1.));
#17190=DIRECTION('ref_axis',(-0.707106781186545,-0.70710678118655,0.));
#17191=DIRECTION('',(0.,0.,-1.));
#17192=DIRECTION('center_axis',(1.,0.,0.));
#17193=DIRECTION('ref_axis',(0.,0.,-1.));
#17194=DIRECTION('center_axis',(1.,0.,0.));
#17195=DIRECTION('ref_axis',(0.,0.,-1.));
#17196=DIRECTION('center_axis',(0.,0.,1.));
#17197=DIRECTION('ref_axis',(0.,1.,0.));
#17198=DIRECTION('center_axis',(1.,0.,0.));
#17199=DIRECTION('ref_axis',(0.,0.707106781186547,0.707106781186547));
#17200=DIRECTION('center_axis',(0.,1.,0.));
#17201=DIRECTION('ref_axis',(-1.,0.,0.));
#17202=DIRECTION('center_axis',(-1.,0.,0.));
#17203=DIRECTION('ref_axis',(0.,0.707106781186548,0.707106781186548));
#17204=DIRECTION('center_axis',(0.,-1.,0.));
#17205=DIRECTION('ref_axis',(-0.707106781186545,0.,0.70710678118655));
#17206=DIRECTION('',(0.,-1.,0.));
#17207=DIRECTION('center_axis',(0.,0.,1.));
#17208=DIRECTION('ref_axis',(-0.707106781186545,0.70710678118655,0.));
#17209=DIRECTION('',(0.,0.,1.));
#17210=DIRECTION('center_axis',(1.,0.,0.));
#17211=DIRECTION('ref_axis',(0.,0.,-1.));
#17212=DIRECTION('center_axis',(0.,1.,0.));
#17213=DIRECTION('ref_axis',(-0.707106781186545,0.,-0.70710678118655));
#17214=DIRECTION('',(0.,1.,0.));
#17215=DIRECTION('center_axis',(0.,-1.,2.22044604925031E-15));
#17216=DIRECTION('ref_axis',(-1.,0.,0.));
#17217=DIRECTION('center_axis',(1.,0.,0.));
#17218=DIRECTION('ref_axis',(0.,0.,-1.));
#17219=DIRECTION('center_axis',(0.,0.,-1.));
#17220=DIRECTION('ref_axis',(-1.,0.,0.));
#17221=DIRECTION('center_axis',(-1.,0.,0.));
#17222=DIRECTION('ref_axis',(0.,0.707106781186548,-0.707106781186548));
#17223=DIRECTION('center_axis',(1.,0.,0.));
#17224=DIRECTION('ref_axis',(0.,0.707106781186547,-0.707106781186547));
#17225=DIRECTION('center_axis',(0.,0.,1.));
#17226=DIRECTION('ref_axis',(-0.707106781186545,0.70710678118655,0.));
#17227=DIRECTION('',(0.,0.,1.));
#17228=DIRECTION('center_axis',(1.,0.,0.));
#17229=DIRECTION('ref_axis',(0.,0.,-1.));
#17230=DIRECTION('center_axis',(0.,0.,-1.));
#17231=DIRECTION('ref_axis',(-0.707106781186545,-0.70710678118655,0.));
#17232=DIRECTION('',(0.,0.,-1.));
#17233=DIRECTION('center_axis',(0.,2.22044604925031E-15,1.));
#17234=DIRECTION('ref_axis',(-1.,0.,0.));
#17235=DIRECTION('center_axis',(1.,0.,0.));
#17236=DIRECTION('ref_axis',(0.,0.,-1.));
#17237=DIRECTION('center_axis',(0.,-1.,0.));
#17238=DIRECTION('ref_axis',(-1.,0.,0.));
#17239=DIRECTION('center_axis',(-1.,0.,0.));
#17240=DIRECTION('ref_axis',(0.,-0.707106781186548,-0.707106781186548));
#17241=DIRECTION('center_axis',(1.,0.,0.));
#17242=DIRECTION('ref_axis',(0.,-0.707106781186547,-0.707106781186547));
#17243=DIRECTION('center_axis',(0.,1.,0.));
#17244=DIRECTION('ref_axis',(-0.707106781186545,0.,-0.70710678118655));
#17245=DIRECTION('',(0.,1.,0.));
#17246=DIRECTION('center_axis',(1.,0.,0.));
#17247=DIRECTION('ref_axis',(0.,0.,-1.));
#17248=DIRECTION('center_axis',(0.,1.,0.));
#17249=DIRECTION('ref_axis',(0.707106781186544,0.,-0.707106781186551));
#17250=DIRECTION('center_axis',(0.,1.,0.));
#17251=DIRECTION('ref_axis',(1.,0.,0.));
#17252=DIRECTION('center_axis',(0.,-1.,2.22044604925031E-15));
#17253=DIRECTION('ref_axis',(0.,-2.22044604925031E-15,-1.));
#17254=DIRECTION('center_axis',(1.,0.,0.));
#17255=DIRECTION('ref_axis',(0.,0.,-1.));
#17256=DIRECTION('center_axis',(0.,0.,-1.));
#17257=DIRECTION('ref_axis',(0.,1.,0.));
#17258=DIRECTION('center_axis',(1.,0.,0.));
#17259=DIRECTION('ref_axis',(0.,0.707106781186548,-0.707106781186548));
#17260=DIRECTION('center_axis',(0.,0.,1.));
#17261=DIRECTION('ref_axis',(0.707106781186544,0.707106781186551,0.));
#17262=DIRECTION('center_axis',(0.,-2.22044604925031E-15,-1.));
#17263=DIRECTION('ref_axis',(0.,1.,-2.22044604925031E-15));
#17264=DIRECTION('center_axis',(1.,0.,0.));
#17265=DIRECTION('ref_axis',(0.,0.,-1.));
#17266=DIRECTION('center_axis',(0.,1.,0.));
#17267=DIRECTION('ref_axis',(0.,0.,1.));
#17268=DIRECTION('center_axis',(1.,0.,0.));
#17269=DIRECTION('ref_axis',(0.,0.707106781186548,0.707106781186548));
#17270=DIRECTION('center_axis',(0.,-1.,0.));
#17271=DIRECTION('ref_axis',(0.707106781186544,0.,0.707106781186551));
#17272=DIRECTION('center_axis',(0.,1.,-2.22044604925031E-15));
#17273=DIRECTION('ref_axis',(0.,2.22044604925031E-15,1.));
#17274=DIRECTION('center_axis',(1.,0.,0.));
#17275=DIRECTION('ref_axis',(0.,0.,-1.));
#17276=DIRECTION('center_axis',(0.,0.,1.));
#17277=DIRECTION('ref_axis',(0.,-1.,0.));
#17278=DIRECTION('center_axis',(1.,0.,0.));
#17279=DIRECTION('ref_axis',(0.,-0.707106781186548,0.707106781186548));
#17280=DIRECTION('center_axis',(0.,0.,-1.));
#17281=DIRECTION('ref_axis',(0.707106781186544,-0.707106781186551,0.));
#17282=DIRECTION('center_axis',(0.,2.22044604925031E-15,1.));
#17283=DIRECTION('ref_axis',(0.,-1.,2.22044604925031E-15));
#17284=DIRECTION('center_axis',(1.,0.,0.));
#17285=DIRECTION('ref_axis',(0.,0.,-1.));
#17286=DIRECTION('center_axis',(1.,0.,0.));
#17287=DIRECTION('ref_axis',(0.,-0.707106781186548,-0.707106781186548));
#17288=DIRECTION('center_axis',(1.,0.,0.));
#17289=DIRECTION('ref_axis',(0.,1.,1.58603289232165E-16));
#17290=DIRECTION('center_axis',(1.,0.,0.));
#17291=DIRECTION('ref_axis',(0.,1.58603289232165E-16,-1.));
#17292=DIRECTION('center_axis',(-1.,0.,0.));
#17293=DIRECTION('ref_axis',(0.,0.,1.));
#17294=DIRECTION('center_axis',(0.,-1.,1.22464679914735E-16));
#17295=DIRECTION('ref_axis',(0.,-1.22464679914735E-16,-1.));
#17296=DIRECTION('center_axis',(-1.,0.,0.));
#17297=DIRECTION('ref_axis',(0.,1.,0.));
#17298=DIRECTION('center_axis',(-1.,0.,0.));
#17299=DIRECTION('ref_axis',(0.,1.,0.));
#17300=DIRECTION('center_axis',(1.,0.,0.));
#17301=DIRECTION('ref_axis',(0.,1.,0.));
#17302=DIRECTION('center_axis',(1.,0.,0.));
#17303=DIRECTION('ref_axis',(0.,0.,-1.));
#17304=DIRECTION('',(1.,0.,0.));
#17305=DIRECTION('center_axis',(-0.518601214467743,-0.756360525034703,0.39871234809297));
#17306=DIRECTION('ref_axis',(0.,-0.466321371218455,-0.884615384641789));
#17307=DIRECTION('center_axis',(-0.518601214553226,0.756360524966231,-0.398712348111676));
#17308=DIRECTION('ref_axis',(0.,-0.466321371268611,-0.884615384615349));
#17309=DIRECTION('center_axis',(0.518601214467742,-0.756360525034697,-0.398712348092983));
#17310=DIRECTION('ref_axis',(4.44089209850065E-15,-0.466321371218468,0.884615384641782));
#17311=DIRECTION('center_axis',(0.518601214552952,0.756360524966382,0.398712348111745));
#17312=DIRECTION('ref_axis',(0.,-0.466321371268601,0.884615384615355));
#17313=DIRECTION('center_axis',(0.,0.,1.));
#17314=DIRECTION('ref_axis',(1.,0.,0.));
#17315=DIRECTION('center_axis',(0.,0.,1.));
#17316=DIRECTION('ref_axis',(1.,0.,0.));
#17317=DIRECTION('',(0.,0.,1.));
#17318=DIRECTION('center_axis',(1.,0.,0.));
#17319=DIRECTION('ref_axis',(0.,0.,-1.));
#17320=DIRECTION('center_axis',(1.,0.,0.));
#17321=DIRECTION('ref_axis',(0.,0.,-1.));
#17322=DIRECTION('center_axis',(1.,0.,0.));
#17323=DIRECTION('ref_axis',(0.,0.,-1.));
#17324=DIRECTION('center_axis',(1.,0.,0.));
#17325=DIRECTION('ref_axis',(0.,0.,-1.));
#17326=DIRECTION('center_axis',(1.,0.,0.));
#17327=DIRECTION('ref_axis',(0.,1.,0.));
#17328=DIRECTION('center_axis',(1.,0.,0.));
#17329=DIRECTION('ref_axis',(0.,1.,0.));
#17330=DIRECTION('',(1.,0.,0.));
#17331=DIRECTION('center_axis',(1.,0.,0.));
#17332=DIRECTION('ref_axis',(0.,0.,-1.));
#17333=DIRECTION('center_axis',(-1.,0.,0.));
#17334=DIRECTION('ref_axis',(0.,0.,1.));
#17335=DIRECTION('center_axis',(1.,0.,0.));
#17336=DIRECTION('ref_axis',(0.,0.,-1.));
#17337=DIRECTION('center_axis',(1.,0.,0.));
#17338=DIRECTION('ref_axis',(0.,1.,0.));
#17339=DIRECTION('',(1.,0.,0.));
#17340=DIRECTION('center_axis',(1.,0.,0.));
#17341=DIRECTION('ref_axis',(0.,0.,-1.));
#17342=DIRECTION('center_axis',(1.,0.,0.));
#17343=DIRECTION('ref_axis',(0.,0.,-1.));
#17344=DIRECTION('center_axis',(1.,0.,0.));
#17345=DIRECTION('ref_axis',(0.,0.,-1.));
#17346=DIRECTION('center_axis',(1.,0.,0.));
#17347=DIRECTION('ref_axis',(0.,1.,0.));
#17348=DIRECTION('',(1.,0.,0.));
#17349=DIRECTION('center_axis',(1.,0.,0.));
#17350=DIRECTION('ref_axis',(0.,0.,-1.));
#17351=DIRECTION('center_axis',(-1.,0.,0.));
#17352=DIRECTION('ref_axis',(0.,0.,1.));
#17353=DIRECTION('center_axis',(-1.,0.,0.));
#17354=DIRECTION('ref_axis',(0.,0.,1.));
#17355=DIRECTION('center_axis',(1.,0.,0.));
#17356=DIRECTION('ref_axis',(0.,-1.58603289232165E-16,1.));
#17357=DIRECTION('center_axis',(1.,0.,0.));
#17358=DIRECTION('ref_axis',(0.,-1.,-1.58603289232165E-16));
#17359=DIRECTION('center_axis',(1.,0.,0.));
#17360=DIRECTION('ref_axis',(0.,0.,-1.));
#17361=DIRECTION('center_axis',(1.,0.,0.));
#17362=DIRECTION('ref_axis',(0.,0.,-1.));
#20891=CARTESIAN_POINT('',(0.,0.,0.));
#20892=CARTESIAN_POINT('Origin',(62.5,18.,-63.75));
#20893=CARTESIAN_POINT('',(48.,18.,-64.));
#20894=CARTESIAN_POINT('Origin',(62.5,18.,-64.));
#20895=CARTESIAN_POINT('',(47.5,18.,-63.5));
#20896=CARTESIAN_POINT('',(47.75,18.,-63.75));
#20897=CARTESIAN_POINT('Origin',(62.5,18.,-63.5));
#20898=CARTESIAN_POINT('Origin',(62.5,18.,-50.));
#20899=CARTESIAN_POINT('',(47.5,18.,-60.));
#20900=CARTESIAN_POINT('',(47.5,18.,-50.));
#20901=CARTESIAN_POINT('',(57.1148351928655,32.,-60.));
#20902=CARTESIAN_POINT('Origin',(62.5,18.,-60.));
#20903=CARTESIAN_POINT('',(67.8851648071345,32.,-60.));
#20904=CARTESIAN_POINT('Ctrl Pts',(67.8851648071345,32.,-60.));
#20905=CARTESIAN_POINT('Ctrl Pts',(67.6984748326239,32.0718111628985,-60.));
#20906=CARTESIAN_POINT('Ctrl Pts',(67.5101785201311,32.1399502129255,-59.9997241719152));
#20907=CARTESIAN_POINT('Ctrl Pts',(65.73704131346,32.7417106379464,-59.9953335785546));
#20908=CARTESIAN_POINT('Ctrl Pts',(64.0583526295515,33.,-59.9821371592664));
#20909=CARTESIAN_POINT('Ctrl Pts',(60.9416473704485,33.,-59.9821371592664));
#20910=CARTESIAN_POINT('Ctrl Pts',(59.26295868654,32.7417106379464,-59.9953335785546));
#20911=CARTESIAN_POINT('Ctrl Pts',(57.4898214798689,32.1399502129255,-59.9997241719152));
#20912=CARTESIAN_POINT('Ctrl Pts',(57.3015251673761,32.0718111628985,-60.));
#20913=CARTESIAN_POINT('Ctrl Pts',(57.1148351928655,32.,-60.));
#20914=CARTESIAN_POINT('Origin',(62.5,18.,-60.));
#20915=CARTESIAN_POINT('Origin',(62.5,18.,-64.));
#20916=CARTESIAN_POINT('',(53.45,18.,-64.));
#20917=CARTESIAN_POINT('Origin',(62.5,18.,-64.));
#20918=CARTESIAN_POINT('Origin',(15.75,-73.,0.));
#20919=CARTESIAN_POINT('',(16.,-73.,7.65));
#20920=CARTESIAN_POINT('Origin',(16.,-73.,0.));
#20921=CARTESIAN_POINT('',(15.5,-73.,7.15));
#20922=CARTESIAN_POINT('',(15.75,-73.,7.4));
#20923=CARTESIAN_POINT('Origin',(15.5,-73.,0.));
#20924=CARTESIAN_POINT('Origin',(16.,0.,0.));
#20925=CARTESIAN_POINT('',(16.,-60.8276253029822,-12.));
#20926=CARTESIAN_POINT('',(16.,-73.,-12.));
#20927=CARTESIAN_POINT('',(16.,-36.5,-12.));
#20928=CARTESIAN_POINT('',(16.,-60.,-15.6204993518133));
#20929=CARTESIAN_POINT('Origin',(16.,0.,0.));
#20930=CARTESIAN_POINT('',(16.,-60.,15.6204993518133));
#20931=CARTESIAN_POINT('',(16.,-60.,16.));
#20932=CARTESIAN_POINT('',(16.,-60.8276253029822,12.));
#20933=CARTESIAN_POINT('Origin',(16.,0.,0.));
#20934=CARTESIAN_POINT('',(16.,-73.,12.));
#20935=CARTESIAN_POINT('',(16.,-30.4559107563704,12.));
#20936=CARTESIAN_POINT('Origin',(16.,-73.,0.));
#20937=CARTESIAN_POINT('Origin',(-0.1,-73.,0.));
#20938=CARTESIAN_POINT('',(0.5,-73.,7.15));
#20939=CARTESIAN_POINT('Origin',(0.5,-73.,0.));
#20940=CARTESIAN_POINT('',(-0.1,-73.,7.15));
#20941=CARTESIAN_POINT('Origin',(62.5,18.,63.75));
#20942=CARTESIAN_POINT('',(48.,18.,64.));
#20943=CARTESIAN_POINT('Origin',(62.5,18.,64.));
#20944=CARTESIAN_POINT('',(47.5,18.,63.5));
#20945=CARTESIAN_POINT('',(47.75,18.,63.75));
#20946=CARTESIAN_POINT('Origin',(62.5,18.,63.5));
#20947=CARTESIAN_POINT('Origin',(62.5,18.,64.));
#20948=CARTESIAN_POINT('',(52.95,18.,64.));
#20949=CARTESIAN_POINT('Origin',(62.5,18.,64.));
#20950=CARTESIAN_POINT('Origin',(62.5,18.,50.));
#20951=CARTESIAN_POINT('',(47.5,18.,60.));
#20952=CARTESIAN_POINT('',(47.5,18.,50.));
#20953=CARTESIAN_POINT('',(67.8851648071345,32.,60.));
#20954=CARTESIAN_POINT('Origin',(62.5,18.,60.));
#20955=CARTESIAN_POINT('',(57.1148351928655,32.,60.));
#20956=CARTESIAN_POINT('Ctrl Pts',(57.1148351928655,32.,60.));
#20957=CARTESIAN_POINT('Ctrl Pts',(57.3015251673761,32.0718111628985,60.));
#20958=CARTESIAN_POINT('Ctrl Pts',(57.4898214798689,32.1399502129255,59.9997241719152));
#20959=CARTESIAN_POINT('Ctrl Pts',(59.26295868654,32.7417106379464,59.9953335785546));
#20960=CARTESIAN_POINT('Ctrl Pts',(60.9416473704485,33.,59.9821371592664));
#20961=CARTESIAN_POINT('Ctrl Pts',(64.0583526295515,33.,59.9821371592664));
#20962=CARTESIAN_POINT('Ctrl Pts',(65.73704131346,32.7417106379464,59.9953335785546));
#20963=CARTESIAN_POINT('Ctrl Pts',(67.5101785201311,32.1399502129255,59.9997241719152));
#20964=CARTESIAN_POINT('Ctrl Pts',(67.6984748326239,32.0718111628985,60.));
#20965=CARTESIAN_POINT('Ctrl Pts',(67.8851648071345,32.,60.));
#20966=CARTESIAN_POINT('Origin',(62.5,18.,60.));
#20967=CARTESIAN_POINT('Origin',(15.75,73.,0.));
#20968=CARTESIAN_POINT('',(16.,73.,7.65));
#20969=CARTESIAN_POINT('Origin',(16.,73.,0.));
#20970=CARTESIAN_POINT('',(15.5,73.,7.15));
#20971=CARTESIAN_POINT('',(15.75,73.,7.4));
#20972=CARTESIAN_POINT('Origin',(15.5,73.,0.));
#20973=CARTESIAN_POINT('Origin',(16.,0.,0.));
#20974=CARTESIAN_POINT('',(16.,73.,-12.));
#20975=CARTESIAN_POINT('',(16.,60.8276253029822,-12.));
#20976=CARTESIAN_POINT('',(16.,30.4559107563704,-12.));
#20977=CARTESIAN_POINT('',(16.,73.,12.));
#20978=CARTESIAN_POINT('Origin',(16.,73.,0.));
#20979=CARTESIAN_POINT('',(16.,60.8276253029822,12.));
#20980=CARTESIAN_POINT('',(16.,36.5,12.));
#20981=CARTESIAN_POINT('',(16.,60.,15.6204993518133));
#20982=CARTESIAN_POINT('Origin',(16.,0.,0.));
#20983=CARTESIAN_POINT('',(16.,60.,-15.6204993518133));
#20984=CARTESIAN_POINT('',(16.,60.,-16.));
#20985=CARTESIAN_POINT('Origin',(16.,0.,0.));
#20986=CARTESIAN_POINT('Origin',(-0.1,73.,0.));
#20987=CARTESIAN_POINT('',(0.5,73.,7.15));
#20988=CARTESIAN_POINT('Origin',(0.5,73.,0.));
#20989=CARTESIAN_POINT('',(-0.1,73.,7.15));
#20990=CARTESIAN_POINT('Origin',(62.5,18.,63.75));
#20991=CARTESIAN_POINT('',(53.45,18.,63.5));
#20992=CARTESIAN_POINT('',(53.2,18.,63.75));
#20993=CARTESIAN_POINT('Origin',(62.5,18.,63.5));
#20994=CARTESIAN_POINT('Origin',(62.5,18.,64.));
#20995=CARTESIAN_POINT('',(53.44935360134,18.0005320189151,48.7866812026286));
#20996=CARTESIAN_POINT('',(53.45,18.,64.));
#20997=CARTESIAN_POINT('',(55.0359921611649,23.1177228316711,46.0000000008449));
#20998=CARTESIAN_POINT('Ctrl Pts',(55.0359921613628,23.1177228319597,46.0000000015041));
#20999=CARTESIAN_POINT('Ctrl Pts',(54.0296627121601,21.6500288704652,46.9446698142113));
#21000=CARTESIAN_POINT('Ctrl Pts',(53.4516146271291,19.8715344775383,47.9435639657356));
#21001=CARTESIAN_POINT('Ctrl Pts',(53.4492786369557,18.0256888439599,48.7753807839716));
#21002=CARTESIAN_POINT('Ctrl Pts',(53.44935360134,18.0005320189151,48.7866812026286));
#21003=CARTESIAN_POINT('',(69.9640078370496,23.1177228342753,46.0000000000068));
#21004=CARTESIAN_POINT('Origin',(62.5,18.,46.));
#21005=CARTESIAN_POINT('Ctrl Pts',(53.44935360134,18.0005320189151,48.7866812026286));
#21006=CARTESIAN_POINT('Ctrl Pts',(53.4547065835389,16.2041584743725,49.5936102599095));
#21007=CARTESIAN_POINT('Ctrl Pts',(54.5621164439011,12.4685238830907,50.8988378408999));
#21008=CARTESIAN_POINT('Ctrl Pts',(59.4315484638286,8.79278472652513,51.5632592674646));
#21009=CARTESIAN_POINT('Ctrl Pts',(65.5663223673701,8.80057359018861,51.5646626464224));
#21010=CARTESIAN_POINT('Ctrl Pts',(70.463129301692,12.4814952571317,50.8974409168532));
#21011=CARTESIAN_POINT('Ctrl Pts',(72.1120278968484,18.1410701930242,48.9161444008817));
#21012=CARTESIAN_POINT('Ctrl Pts',(70.9703446072329,21.6500181963829,46.944676684654));
#21013=CARTESIAN_POINT('Ctrl Pts',(69.964007837035,23.1177228342965,46.));
#21014=CARTESIAN_POINT('Origin',(125.55,45.,-45.));
#21015=CARTESIAN_POINT('',(125.8,45.,-38.45));
#21016=CARTESIAN_POINT('Origin',(125.8,45.,-45.));
#21017=CARTESIAN_POINT('',(125.3,45.,-38.95));
#21018=CARTESIAN_POINT('',(125.55,45.,-38.7));
#21019=CARTESIAN_POINT('Origin',(125.3,45.,-45.));
#21020=CARTESIAN_POINT('Origin',(125.8,0.,0.));
#21021=CARTESIAN_POINT('',(125.8,32.,-58.));
#21022=CARTESIAN_POINT('',(125.8,-32.,-58.));
#21023=CARTESIAN_POINT('',(125.8,-16.,-58.));
#21024=CARTESIAN_POINT('',(125.8,58.,-32.));
#21025=CARTESIAN_POINT('Origin',(125.8,32.,-32.));
#21026=CARTESIAN_POINT('',(125.8,58.,32.));
#21027=CARTESIAN_POINT('',(125.8,58.,-16.));
#21028=CARTESIAN_POINT('',(125.8,32.,58.));
#21029=CARTESIAN_POINT('Origin',(125.8,32.,32.));
#21030=CARTESIAN_POINT('',(125.8,-32.,58.));
#21031=CARTESIAN_POINT('',(125.8,16.,58.));
#21032=CARTESIAN_POINT('',(125.8,-58.,32.));
#21033=CARTESIAN_POINT('Origin',(125.8,-32.,32.));
#21034=CARTESIAN_POINT('',(125.8,-58.,-32.));
#21035=CARTESIAN_POINT('',(125.8,-58.,16.));
#21036=CARTESIAN_POINT('Origin',(125.8,-32.,-32.));
#21037=CARTESIAN_POINT('',(125.8,-45.,51.55));
#21038=CARTESIAN_POINT('Origin',(125.8,-45.,45.));
#21039=CARTESIAN_POINT('',(125.8,-45.,-38.45));
#21040=CARTESIAN_POINT('Origin',(125.8,-45.,-45.));
#21041=CARTESIAN_POINT('',(125.8,-6.36816335556624E-15,-52.));
#21042=CARTESIAN_POINT('Origin',(125.8,0.,0.));
#21043=CARTESIAN_POINT('',(125.8,45.,51.55));
#21044=CARTESIAN_POINT('Origin',(125.8,45.,45.));
#21045=CARTESIAN_POINT('Origin',(125.8,45.,-45.));
#21046=CARTESIAN_POINT('',(99.8,45.,-38.95));
#21047=CARTESIAN_POINT('',(125.8,45.,-38.95));
#21048=CARTESIAN_POINT('Origin',(99.8,45.,-45.));
#21049=CARTESIAN_POINT('Origin',(125.55,-45.,45.));
#21050=CARTESIAN_POINT('',(125.3,-45.,51.05));
#21051=CARTESIAN_POINT('',(125.55,-45.,51.3));
#21052=CARTESIAN_POINT('Origin',(125.3,-45.,45.));
#21053=CARTESIAN_POINT('Origin',(125.8,-45.,45.));
#21054=CARTESIAN_POINT('',(99.8,-45.,51.05));
#21055=CARTESIAN_POINT('',(125.8,-45.,51.05));
#21056=CARTESIAN_POINT('Origin',(99.8,-45.,45.));
#21057=CARTESIAN_POINT('Origin',(125.55,45.,45.));
#21058=CARTESIAN_POINT('',(125.3,45.,51.05));
#21059=CARTESIAN_POINT('',(125.55,45.,51.3));
#21060=CARTESIAN_POINT('Origin',(125.3,45.,45.));
#21061=CARTESIAN_POINT('Origin',(125.8,45.,45.));
#21062=CARTESIAN_POINT('',(99.8,45.,51.05));
#21063=CARTESIAN_POINT('',(125.8,45.,51.05));
#21064=CARTESIAN_POINT('Origin',(99.8,45.,45.));
#21065=CARTESIAN_POINT('Origin',(125.55,-45.,-45.));
#21066=CARTESIAN_POINT('',(125.3,-45.,-38.95));
#21067=CARTESIAN_POINT('',(125.55,-45.,-38.7));
#21068=CARTESIAN_POINT('Origin',(125.3,-45.,-45.));
#21069=CARTESIAN_POINT('Origin',(125.8,-45.,-45.));
#21070=CARTESIAN_POINT('',(99.8,-45.,-38.95));
#21071=CARTESIAN_POINT('',(125.8,-45.,-38.95));
#21072=CARTESIAN_POINT('Origin',(99.8,-45.,-45.));
#21073=CARTESIAN_POINT('Origin',(15.75,0.,0.));
#21074=CARTESIAN_POINT('',(15.4999999969433,-61.0634996055951,-13.3228756624643));
#21075=CARTESIAN_POINT('Ctrl Pts',(15.4999999966277,-61.0634996097249,-13.3228756593561));
#21076=CARTESIAN_POINT('Ctrl Pts',(15.5800859964154,-61.0013423773347,-13.2320666717072));
#21077=CARTESIAN_POINT('Ctrl Pts',(15.6534629211121,-60.9478909731446,-13.1321977587055));
#21078=CARTESIAN_POINT('Ctrl Pts',(15.8336779042045,-60.8282401952317,-12.8299273372329));
#21079=CARTESIAN_POINT('Ctrl Pts',(15.9261070025809,-60.7835362526876,-12.5931700844189));
#21080=CARTESIAN_POINT('Ctrl Pts',(15.9898935814354,-60.7916707113854,-12.2327047392017));
#21081=CARTESIAN_POINT('Ctrl Pts',(16.,-60.80493204889,-12.1150313964023));
#21082=CARTESIAN_POINT('Ctrl Pts',(16.,-60.8276253029822,-11.9999999999999));
#21083=CARTESIAN_POINT('',(15.5,-59.8580811200045,-17.9794361599846));
#21084=CARTESIAN_POINT('Origin',(15.5,0.,0.));
#21085=CARTESIAN_POINT('',(15.6381526893245,-60.,-17.));
#21086=CARTESIAN_POINT('Ctrl Pts',(15.5,-59.8580811200045,-17.9794361599846));
#21087=CARTESIAN_POINT('Ctrl Pts',(15.5485606843564,-59.9053376415118,-17.6533009342783));
#21088=CARTESIAN_POINT('Ctrl Pts',(15.5946215988532,-59.9526427924876,-17.3268300981166));
#21089=CARTESIAN_POINT('Ctrl Pts',(15.6381526893245,-60.,-17.));
#21090=CARTESIAN_POINT('Ctrl Pts',(15.6381526893245,-60.,-17.));
#21091=CARTESIAN_POINT('Ctrl Pts',(15.826727493626,-60.,-16.3082427557362));
#21092=CARTESIAN_POINT('Ctrl Pts',(16.,-60.,-15.6204993518134));
#21093=CARTESIAN_POINT('Origin',(0.,-59.9290405600022,-17.4897180799923));
#21094=CARTESIAN_POINT('',(17.2600442058128,-59.858081116524,-17.9794361715722));
#21095=CARTESIAN_POINT('',(0.,-59.8580811200045,-17.9794361599846));
#21096=CARTESIAN_POINT('',(18.,-60.,-17.));
#21097=CARTESIAN_POINT('Origin',(18.,-58.,-30.8027605631545));
#21098=CARTESIAN_POINT('',(0.,-60.,-17.));
#21099=CARTESIAN_POINT('Origin',(16.,-60.,32.));
#21100=CARTESIAN_POINT('',(18.,-60.,-32.));
#21101=CARTESIAN_POINT('',(18.,-60.,16.));
#21102=CARTESIAN_POINT('',(123.8,-60.,-32.));
#21103=CARTESIAN_POINT('',(16.,-60.,-32.));
#21104=CARTESIAN_POINT('',(123.8,-60.,32.));
#21105=CARTESIAN_POINT('',(123.8,-60.,16.));
#21106=CARTESIAN_POINT('',(18.,-60.,32.));
#21107=CARTESIAN_POINT('',(16.,-60.,32.));
#21108=CARTESIAN_POINT('',(18.,-60.,17.));
#21109=CARTESIAN_POINT('',(18.,-60.,16.));
#21110=CARTESIAN_POINT('',(15.6381526893245,-60.,17.));
#21111=CARTESIAN_POINT('',(0.,-60.,17.));
#21112=CARTESIAN_POINT('Ctrl Pts',(16.,-60.,15.6204993518133));
#21113=CARTESIAN_POINT('Ctrl Pts',(15.826727493626,-60.,16.3082427557361));
#21114=CARTESIAN_POINT('Ctrl Pts',(15.6381526893245,-60.,17.));
#21115=CARTESIAN_POINT('Origin',(0.,-17.4897180799923,-59.9290405600022));
#21116=CARTESIAN_POINT('',(14.,-17.9794361599846,-59.8580811200045));
#21117=CARTESIAN_POINT('',(14.7304276784111,-16.9999999991831,-60.));
#21118=CARTESIAN_POINT('Ctrl Pts',(14.7304276776349,-16.9999999989424,-60.0000000001532));
#21119=CARTESIAN_POINT('Ctrl Pts',(14.6761902161882,-17.159755202079,-59.9768517027666));
#21120=CARTESIAN_POINT('Ctrl Pts',(14.6152171518727,-17.3169819821409,-59.9540697702187));
#21121=CARTESIAN_POINT('Ctrl Pts',(14.4632746479611,-17.6188900437764,-59.9103237296707));
#21122=CARTESIAN_POINT('Ctrl Pts',(14.3588395089388,-17.7908531163461,-59.8854065296971));
#21123=CARTESIAN_POINT('Ctrl Pts',(14.1914653455901,-17.9195593830331,-59.8667571781999));
#21124=CARTESIAN_POINT('Ctrl Pts',(14.1471388512752,-17.9457470523029,-59.8629626228789));
#21125=CARTESIAN_POINT('Ctrl Pts',(14.074547869931,-17.9718483805388,-59.8591805782485));
#21126=CARTESIAN_POINT('Ctrl Pts',(14.0342136843971,-17.9794361599847,-59.8580811200045));
#21127=CARTESIAN_POINT('Ctrl Pts',(14.,-17.9794361599847,-59.8580811200045));
#21128=CARTESIAN_POINT('',(18.,-17.,-60.));
#21129=CARTESIAN_POINT('',(0.,-17.,-60.));
#21130=CARTESIAN_POINT('',(17.2600442058128,-17.9794361715722,-59.858081116524));
#21131=CARTESIAN_POINT('Origin',(18.,-30.8027605631545,-58.));
#21132=CARTESIAN_POINT('',(0.,-17.9794361599846,-59.8580811200045));
#21133=CARTESIAN_POINT('Origin',(16.,-32.,-60.));
#21134=CARTESIAN_POINT('',(18.,-32.,-60.));
#21135=CARTESIAN_POINT('',(18.,-16.,-60.));
#21136=CARTESIAN_POINT('',(16.,-7.76208734813001,-60.));
#21137=CARTESIAN_POINT('Ctrl Pts',(14.7304276780283,-16.9999999989171,-60.));
#21138=CARTESIAN_POINT('Ctrl Pts',(14.8398686953361,-16.8424989931707,-60.));
#21139=CARTESIAN_POINT('Ctrl Pts',(14.9313718498422,-16.6679371205732,-60.));
#21140=CARTESIAN_POINT('Ctrl Pts',(15.2970561697214,-15.8666064940819,-60.));
#21141=CARTESIAN_POINT('Ctrl Pts',(15.4592365878721,-15.1702769231182,-60.));
#21142=CARTESIAN_POINT('Ctrl Pts',(15.7175697501628,-13.7281199101031,-60.));
#21143=CARTESIAN_POINT('Ctrl Pts',(15.8016080012342,-12.9801486404093,-60.));
#21144=CARTESIAN_POINT('Ctrl Pts',(15.9799340791093,-10.7101781630257,-60.));
#21145=CARTESIAN_POINT('Ctrl Pts',(16.,-9.16876356419723,-60.));
#21146=CARTESIAN_POINT('Ctrl Pts',(16.,-7.76208734813001,-60.));
#21147=CARTESIAN_POINT('',(16.,7.76208734813001,-60.));
#21148=CARTESIAN_POINT('',(16.,-16.,-60.));
#21149=CARTESIAN_POINT('',(14.7304276784111,16.9999999991831,-60.));
#21150=CARTESIAN_POINT('Ctrl Pts',(16.,7.76208734813,-60.));
#21151=CARTESIAN_POINT('Ctrl Pts',(16.,9.16876356419723,-60.));
#21152=CARTESIAN_POINT('Ctrl Pts',(15.9799340791093,10.7101781630257,-60.));
#21153=CARTESIAN_POINT('Ctrl Pts',(15.8016080012342,12.9801486404093,-60.));
#21154=CARTESIAN_POINT('Ctrl Pts',(15.7175697501628,13.7281199101031,-60.));
#21155=CARTESIAN_POINT('Ctrl Pts',(15.4592365878721,15.1702769231182,-60.));
#21156=CARTESIAN_POINT('Ctrl Pts',(15.2970561697214,15.8666064940819,-60.));
#21157=CARTESIAN_POINT('Ctrl Pts',(14.9313718498422,16.6679371205732,-60.));
#21158=CARTESIAN_POINT('Ctrl Pts',(14.8398686953361,16.8424989931707,-60.));
#21159=CARTESIAN_POINT('Ctrl Pts',(14.7304276780283,16.9999999989171,-60.));
#21160=CARTESIAN_POINT('',(18.,17.,-60.));
#21161=CARTESIAN_POINT('',(0.,17.,-60.));
#21162=CARTESIAN_POINT('',(18.,32.,-60.));
#21163=CARTESIAN_POINT('',(18.,-16.,-60.));
#21164=CARTESIAN_POINT('',(16.,32.,-60.));
#21165=CARTESIAN_POINT('',(123.8,32.,-60.));
#21166=CARTESIAN_POINT('',(16.,32.,-60.));
#21167=CARTESIAN_POINT('',(123.8,-32.,-60.));
#21168=CARTESIAN_POINT('',(123.8,-16.,-60.));
#21169=CARTESIAN_POINT('',(16.,-32.,-60.));
#21170=CARTESIAN_POINT('Origin',(0.,17.4897180799923,-59.9290405600022));
#21171=CARTESIAN_POINT('',(17.2600442058128,17.9794361715722,-59.858081116524));
#21172=CARTESIAN_POINT('Origin',(18.,30.8027605631545,-58.));
#21173=CARTESIAN_POINT('',(14.,17.9794361599846,-59.8580811200045));
#21174=CARTESIAN_POINT('Ctrl Pts',(14.,17.9794361599847,-59.8580811200045));
#21175=CARTESIAN_POINT('Ctrl Pts',(14.0342136843971,17.9794361599847,-59.8580811200045));
#21176=CARTESIAN_POINT('Ctrl Pts',(14.074547869931,17.9718483805388,-59.8591805782485));
#21177=CARTESIAN_POINT('Ctrl Pts',(14.1471388512752,17.9457470523029,-59.8629626228789));
#21178=CARTESIAN_POINT('Ctrl Pts',(14.1914653455901,17.9195593830331,-59.8667571781999));
#21179=CARTESIAN_POINT('Ctrl Pts',(14.3588395089388,17.7908531163461,-59.8854065296971));
#21180=CARTESIAN_POINT('Ctrl Pts',(14.4632746479611,17.6188900437764,-59.9103237296707));
#21181=CARTESIAN_POINT('Ctrl Pts',(14.6152171518727,17.3169819821409,-59.9540697702187));
#21182=CARTESIAN_POINT('Ctrl Pts',(14.6761902161882,17.159755202079,-59.9768517027666));
#21183=CARTESIAN_POINT('Ctrl Pts',(14.7304276776349,16.9999999989424,-60.0000000001532));
#21184=CARTESIAN_POINT('',(0.,17.9794361599846,-59.8580811200045));
#21185=CARTESIAN_POINT('Origin',(15.75,0.,0.));
#21186=CARTESIAN_POINT('',(15.5,59.8580811200045,-17.9794361599846));
#21187=CARTESIAN_POINT('',(15.4999999969433,61.0634996055951,-13.3228756624643));
#21188=CARTESIAN_POINT('Origin',(15.5,0.,0.));
#21189=CARTESIAN_POINT('Ctrl Pts',(16.,60.8276253029822,-11.9999999999999));
#21190=CARTESIAN_POINT('Ctrl Pts',(16.,60.80493204889,-12.1150313964023));
#21191=CARTESIAN_POINT('Ctrl Pts',(15.9898935814354,60.7916707113854,-12.2327047392017));
#21192=CARTESIAN_POINT('Ctrl Pts',(15.9261070025809,60.7835362526876,-12.5931700844189));
#21193=CARTESIAN_POINT('Ctrl Pts',(15.8336779042045,60.8282401952317,-12.8299273372329));
#21194=CARTESIAN_POINT('Ctrl Pts',(15.6534629211121,60.9478909731446,-13.1321977587055));
#21195=CARTESIAN_POINT('Ctrl Pts',(15.5800859964154,61.0013423773347,-13.2320666717072));
#21196=CARTESIAN_POINT('Ctrl Pts',(15.4999999966277,61.0634996097249,-13.3228756593561));
#21197=CARTESIAN_POINT('',(15.6381526893245,60.,-17.));
#21198=CARTESIAN_POINT('Ctrl Pts',(16.,60.,-15.6204993518133));
#21199=CARTESIAN_POINT('Ctrl Pts',(15.826727493626,60.,-16.3082427557361));
#21200=CARTESIAN_POINT('Ctrl Pts',(15.6381526893245,60.,-17.));
#21201=CARTESIAN_POINT('Ctrl Pts',(15.6381526893245,60.,-17.));
#21202=CARTESIAN_POINT('Ctrl Pts',(15.5946215988532,59.9526427924876,-17.3268300981166));
#21203=CARTESIAN_POINT('Ctrl Pts',(15.5485606843564,59.9053376415118,-17.6533009342783));
#21204=CARTESIAN_POINT('Ctrl Pts',(15.5,59.8580811200045,-17.9794361599846));
#21205=CARTESIAN_POINT('Origin',(0.,59.9290405600022,-17.4897180799923));
#21206=CARTESIAN_POINT('',(18.,60.,-17.));
#21207=CARTESIAN_POINT('',(0.,60.,-17.));
#21208=CARTESIAN_POINT('',(17.2600442058128,59.858081116524,-17.9794361715722));
#21209=CARTESIAN_POINT('Origin',(18.,58.,-30.8027605631545));
#21210=CARTESIAN_POINT('',(0.,59.8580811200045,-17.9794361599846));
#21211=CARTESIAN_POINT('Origin',(0.,0.,0.));
#21212=CARTESIAN_POINT('',(14.,-60.9118215127409,-14.));
#21213=CARTESIAN_POINT('Ctrl Pts',(15.499999995189,-61.0634996059174,-13.3228756609874));
#21214=CARTESIAN_POINT('Ctrl Pts',(15.4701909647076,-61.056125041613,-13.3566759242301));
#21215=CARTESIAN_POINT('Ctrl Pts',(15.4394885037721,-61.0490034120379,-13.3891821198367));
#21216=CARTESIAN_POINT('Ctrl Pts',(15.2319678738428,-61.0037715519876,-13.5949189134652));
#21217=CARTESIAN_POINT('Ctrl Pts',(15.008663619483,-60.9694430253741,-13.7472835331182));
#21218=CARTESIAN_POINT('Ctrl Pts',(14.5181770858478,-60.9234160168088,-13.9498447390067));
#21219=CARTESIAN_POINT('Ctrl Pts',(14.2509679895827,-60.9118215127409,-14.));
#21220=CARTESIAN_POINT('Ctrl Pts',(14.,-60.9118215127409,-14.));
#21221=CARTESIAN_POINT('',(2.,-60.9118215127409,-14.));
#21222=CARTESIAN_POINT('',(0.,-60.9118215127409,-14.));
#21223=CARTESIAN_POINT('',(2.,60.9118215127409,-14.));
#21224=CARTESIAN_POINT('Origin',(2.,0.,0.));
#21225=CARTESIAN_POINT('',(14.,60.9118215127409,-14.));
#21226=CARTESIAN_POINT('',(0.,60.9118215127409,-14.));
#21227=CARTESIAN_POINT('Ctrl Pts',(14.,60.9118215127409,-14.));
#21228=CARTESIAN_POINT('Ctrl Pts',(14.2509679895827,60.9118215127409,-14.));
#21229=CARTESIAN_POINT('Ctrl Pts',(14.5181770858478,60.9234160168088,-13.9498447390067));
#21230=CARTESIAN_POINT('Ctrl Pts',(15.008663619483,60.9694430253741,-13.7472835331182));
#21231=CARTESIAN_POINT('Ctrl Pts',(15.2319678738428,61.0037715519876,-13.5949189134652));
#21232=CARTESIAN_POINT('Ctrl Pts',(15.4394885037721,61.0490034120379,-13.3891821198367));
#21233=CARTESIAN_POINT('Ctrl Pts',(15.4701909647076,61.056125041613,-13.3566759242301));
#21234=CARTESIAN_POINT('Ctrl Pts',(15.499999995189,61.0634996059174,-13.3228756609874));
#21235=CARTESIAN_POINT('',(16.,58.,-23.28626204439));
#21236=CARTESIAN_POINT('Ctrl Pts',(17.2600442115558,59.8580811153305,-17.9794361755454));
#21237=CARTESIAN_POINT('Ctrl Pts',(17.127243690827,59.8051950958716,-18.1555070829828));
#21238=CARTESIAN_POINT('Ctrl Pts',(17.0139600323404,59.7441024880535,-18.3559136759436));
#21239=CARTESIAN_POINT('Ctrl Pts',(16.7810925644696,59.5935235342901,-18.8400023150408));
#21240=CARTESIAN_POINT('Ctrl Pts',(16.6727999393301,59.5012270640763,-19.1293647114412));
#21241=CARTESIAN_POINT('Ctrl Pts',(16.195648993787,59.0240761185332,-20.5909899649672));
#21242=CARTESIAN_POINT('Ctrl Pts',(16.,58.4904260224498,-22.0647388455243));
#21243=CARTESIAN_POINT('Ctrl Pts',(16.,58.,-23.28626204439));
#21244=CARTESIAN_POINT('',(16.,23.28626204439,-58.));
#21245=CARTESIAN_POINT('Origin',(16.,0.,0.));
#21246=CARTESIAN_POINT('Ctrl Pts',(16.,23.28626204439,-58.));
#21247=CARTESIAN_POINT('Ctrl Pts',(16.,22.0647388455243,-58.4904260224498));
#21248=CARTESIAN_POINT('Ctrl Pts',(16.195648993787,20.5909899649672,-59.0240761185332));
#21249=CARTESIAN_POINT('Ctrl Pts',(16.6727999393301,19.1293647114412,-59.5012270640763));
#21250=CARTESIAN_POINT('Ctrl Pts',(16.7810925644696,18.8400023150408,-59.5935235342901));
#21251=CARTESIAN_POINT('Ctrl Pts',(17.0139600323404,18.3559136759436,-59.7441024880535));
#21252=CARTESIAN_POINT('Ctrl Pts',(17.127243690827,18.1555070829828,-59.8051950958716));
#21253=CARTESIAN_POINT('Ctrl Pts',(17.2600442115558,17.9794361755454,-59.8580811153305));
#21254=CARTESIAN_POINT('Origin',(14.,0.,0.));
#21255=CARTESIAN_POINT('',(16.,-23.28626204439,-58.));
#21256=CARTESIAN_POINT('Ctrl Pts',(17.2600442115558,-17.9794361755454,-59.8580811153305));
#21257=CARTESIAN_POINT('Ctrl Pts',(17.127243690827,-18.1555070829828,-59.8051950958716));
#21258=CARTESIAN_POINT('Ctrl Pts',(17.0139600323404,-18.3559136759436,-59.7441024880535));
#21259=CARTESIAN_POINT('Ctrl Pts',(16.7810925644696,-18.8400023150408,-59.5935235342901));
#21260=CARTESIAN_POINT('Ctrl Pts',(16.6727999393301,-19.1293647114412,-59.5012270640763));
#21261=CARTESIAN_POINT('Ctrl Pts',(16.195648993787,-20.5909899649672,-59.0240761185332));
#21262=CARTESIAN_POINT('Ctrl Pts',(16.,-22.0647388455243,-58.4904260224498));
#21263=CARTESIAN_POINT('Ctrl Pts',(16.,-23.28626204439,-58.));
#21264=CARTESIAN_POINT('',(16.,-58.,-23.28626204439));
#21265=CARTESIAN_POINT('Origin',(16.,0.,0.));
#21266=CARTESIAN_POINT('Ctrl Pts',(16.,-58.,-23.28626204439));
#21267=CARTESIAN_POINT('Ctrl Pts',(16.,-58.4904260224498,-22.0647388455243));
#21268=CARTESIAN_POINT('Ctrl Pts',(16.195648993787,-59.0240761185332,-20.5909899649672));
#21269=CARTESIAN_POINT('Ctrl Pts',(16.6727999393301,-59.5012270640763,-19.1293647114412));
#21270=CARTESIAN_POINT('Ctrl Pts',(16.7810925644696,-59.5935235342901,-18.8400023150408));
#21271=CARTESIAN_POINT('Ctrl Pts',(17.0139600323404,-59.7441024880535,-18.3559136759436));
#21272=CARTESIAN_POINT('Ctrl Pts',(17.127243690827,-59.8051950958716,-18.1555070829828));
#21273=CARTESIAN_POINT('Ctrl Pts',(17.2600442115558,-59.8580811153305,-17.9794361755454));
#21274=CARTESIAN_POINT('Origin',(15.75,0.,0.));
#21275=CARTESIAN_POINT('',(15.4999999969433,61.0634996055951,13.3228756624643));
#21276=CARTESIAN_POINT('Ctrl Pts',(15.4999999966277,61.0634996097249,13.3228756593561));
#21277=CARTESIAN_POINT('Ctrl Pts',(15.5800859964154,61.0013423773347,13.2320666717072));
#21278=CARTESIAN_POINT('Ctrl Pts',(15.6534629211121,60.9478909731446,13.1321977587055));
#21279=CARTESIAN_POINT('Ctrl Pts',(15.8336779042045,60.8282401952317,12.8299273372328));
#21280=CARTESIAN_POINT('Ctrl Pts',(15.9261070025809,60.7835362526876,12.5931700844189));
#21281=CARTESIAN_POINT('Ctrl Pts',(15.9898935814354,60.7916707113854,12.2327047392017));
#21282=CARTESIAN_POINT('Ctrl Pts',(16.,60.80493204889,12.1150313964023));
#21283=CARTESIAN_POINT('Ctrl Pts',(16.,60.8276253029822,11.9999999999999));
#21284=CARTESIAN_POINT('',(15.5,59.8580811200045,17.9794361599846));
#21285=CARTESIAN_POINT('Origin',(15.5,0.,0.));
#21286=CARTESIAN_POINT('',(15.6381526893245,60.,17.));
#21287=CARTESIAN_POINT('Ctrl Pts',(15.5,59.8580811200045,17.9794361599846));
#21288=CARTESIAN_POINT('Ctrl Pts',(15.5485606843564,59.9053376415117,17.6533009342786));
#21289=CARTESIAN_POINT('Ctrl Pts',(15.5946215988532,59.9526427924876,17.3268300981168));
#21290=CARTESIAN_POINT('Ctrl Pts',(15.6381526893245,60.,17.));
#21291=CARTESIAN_POINT('Ctrl Pts',(15.6381526893245,60.,17.));
#21292=CARTESIAN_POINT('Ctrl Pts',(15.826727493626,60.,16.3082427557361));
#21293=CARTESIAN_POINT('Ctrl Pts',(16.,60.,15.6204993518132));
#21294=CARTESIAN_POINT('Origin',(0.,59.9290405600022,17.4897180799923));
#21295=CARTESIAN_POINT('',(17.2600442058128,59.858081116524,17.9794361715722));
#21296=CARTESIAN_POINT('',(0.,59.8580811200045,17.9794361599846));
#21297=CARTESIAN_POINT('',(18.,60.,17.));
#21298=CARTESIAN_POINT('Origin',(18.,58.,30.8027605631545));
#21299=CARTESIAN_POINT('',(0.,60.,17.));
#21300=CARTESIAN_POINT('Origin',(16.,60.,-32.));
#21301=CARTESIAN_POINT('',(18.,60.,32.));
#21302=CARTESIAN_POINT('',(18.,60.,-16.));
#21303=CARTESIAN_POINT('',(123.8,60.,32.));
#21304=CARTESIAN_POINT('',(16.,60.,32.));
#21305=CARTESIAN_POINT('',(123.8,60.,-32.));
#21306=CARTESIAN_POINT('',(123.8,60.,-16.));
#21307=CARTESIAN_POINT('',(18.,60.,-32.));
#21308=CARTESIAN_POINT('',(16.,60.,-32.));
#21309=CARTESIAN_POINT('',(18.,60.,-16.));
#21310=CARTESIAN_POINT('Origin',(0.,17.4897180799923,59.9290405600022));
#21311=CARTESIAN_POINT('',(14.,17.9794361599846,59.8580811200045));
#21312=CARTESIAN_POINT('',(14.7304276784111,16.9999999991831,60.));
#21313=CARTESIAN_POINT('Ctrl Pts',(14.7304276776349,16.9999999989424,60.0000000001532));
#21314=CARTESIAN_POINT('Ctrl Pts',(14.6761902161882,17.159755202079,59.9768517027666));
#21315=CARTESIAN_POINT('Ctrl Pts',(14.6152171518727,17.3169819821409,59.9540697702187));
#21316=CARTESIAN_POINT('Ctrl Pts',(14.4632746479611,17.6188900437764,59.9103237296707));
#21317=CARTESIAN_POINT('Ctrl Pts',(14.3588395089388,17.7908531163461,59.8854065296971));
#21318=CARTESIAN_POINT('Ctrl Pts',(14.1914653455901,17.9195593830331,59.8667571781999));
#21319=CARTESIAN_POINT('Ctrl Pts',(14.1471388512752,17.9457470523029,59.8629626228789));
#21320=CARTESIAN_POINT('Ctrl Pts',(14.074547869931,17.9718483805388,59.8591805782485));
#21321=CARTESIAN_POINT('Ctrl Pts',(14.0342136843971,17.9794361599847,59.8580811200045));
#21322=CARTESIAN_POINT('Ctrl Pts',(14.,17.9794361599847,59.8580811200045));
#21323=CARTESIAN_POINT('',(18.,17.,60.));
#21324=CARTESIAN_POINT('',(0.,17.,60.));
#21325=CARTESIAN_POINT('',(17.2600442058128,17.9794361715722,59.858081116524));
#21326=CARTESIAN_POINT('Origin',(18.,30.8027605631545,58.));
#21327=CARTESIAN_POINT('',(0.,17.9794361599846,59.8580811200045));
#21328=CARTESIAN_POINT('Origin',(16.,32.,60.));
#21329=CARTESIAN_POINT('',(18.,32.,60.));
#21330=CARTESIAN_POINT('',(18.,16.,60.));
#21331=CARTESIAN_POINT('',(16.,7.76208734813001,60.));
#21332=CARTESIAN_POINT('Ctrl Pts',(14.7304276780283,16.9999999989171,60.));
#21333=CARTESIAN_POINT('Ctrl Pts',(14.8398686953361,16.8424989931707,60.));
#21334=CARTESIAN_POINT('Ctrl Pts',(14.9313718498422,16.6679371205732,60.));
#21335=CARTESIAN_POINT('Ctrl Pts',(15.2970561697214,15.8666064940819,60.));
#21336=CARTESIAN_POINT('Ctrl Pts',(15.4592365878721,15.1702769231182,60.));
#21337=CARTESIAN_POINT('Ctrl Pts',(15.7175697501628,13.7281199101031,60.));
#21338=CARTESIAN_POINT('Ctrl Pts',(15.8016080012342,12.9801486404093,60.));
#21339=CARTESIAN_POINT('Ctrl Pts',(15.9799340791093,10.7101781630257,60.));
#21340=CARTESIAN_POINT('Ctrl Pts',(16.,9.16876356419723,60.));
#21341=CARTESIAN_POINT('Ctrl Pts',(16.,7.76208734813001,60.));
#21342=CARTESIAN_POINT('',(16.,-7.76208734813001,60.));
#21343=CARTESIAN_POINT('',(16.,16.,60.));
#21344=CARTESIAN_POINT('',(14.7304276784111,-16.9999999991831,60.));
#21345=CARTESIAN_POINT('Ctrl Pts',(16.,-7.76208734813,60.));
#21346=CARTESIAN_POINT('Ctrl Pts',(16.,-9.16876356419723,60.));
#21347=CARTESIAN_POINT('Ctrl Pts',(15.9799340791093,-10.7101781630257,60.));
#21348=CARTESIAN_POINT('Ctrl Pts',(15.8016080012342,-12.9801486404093,60.));
#21349=CARTESIAN_POINT('Ctrl Pts',(15.7175697501628,-13.7281199101031,60.));
#21350=CARTESIAN_POINT('Ctrl Pts',(15.4592365878721,-15.1702769231182,60.));
#21351=CARTESIAN_POINT('Ctrl Pts',(15.2970561697214,-15.8666064940819,60.));
#21352=CARTESIAN_POINT('Ctrl Pts',(14.9313718498422,-16.6679371205732,60.));
#21353=CARTESIAN_POINT('Ctrl Pts',(14.8398686953361,-16.8424989931707,60.));
#21354=CARTESIAN_POINT('Ctrl Pts',(14.7304276780283,-16.9999999989171,60.));
#21355=CARTESIAN_POINT('',(18.,-17.,60.));
#21356=CARTESIAN_POINT('',(0.,-17.,60.));
#21357=CARTESIAN_POINT('',(18.,-32.,60.));
#21358=CARTESIAN_POINT('',(18.,16.,60.));
#21359=CARTESIAN_POINT('',(123.8,-32.,60.));
#21360=CARTESIAN_POINT('',(16.,-32.,60.));
#21361=CARTESIAN_POINT('',(123.8,32.,60.));
#21362=CARTESIAN_POINT('',(123.8,16.,60.));
#21363=CARTESIAN_POINT('',(16.,32.,60.));
#21364=CARTESIAN_POINT('',(16.,32.,60.));
#21365=CARTESIAN_POINT('Origin',(0.,-17.4897180799923,59.9290405600022));
#21366=CARTESIAN_POINT('',(17.2600442058128,-17.9794361715722,59.858081116524));
#21367=CARTESIAN_POINT('Origin',(18.,-30.8027605631545,58.));
#21368=CARTESIAN_POINT('',(14.,-17.9794361599846,59.8580811200045));
#21369=CARTESIAN_POINT('Ctrl Pts',(14.,-17.9794361599847,59.8580811200045));
#21370=CARTESIAN_POINT('Ctrl Pts',(14.0342136843971,-17.9794361599847,59.8580811200045));
#21371=CARTESIAN_POINT('Ctrl Pts',(14.074547869931,-17.9718483805388,59.8591805782485));
#21372=CARTESIAN_POINT('Ctrl Pts',(14.1471388512752,-17.9457470523029,59.8629626228789));
#21373=CARTESIAN_POINT('Ctrl Pts',(14.1914653455901,-17.9195593830331,59.8667571781999));
#21374=CARTESIAN_POINT('Ctrl Pts',(14.3588395089388,-17.7908531163461,59.8854065296971));
#21375=CARTESIAN_POINT('Ctrl Pts',(14.4632746479611,-17.6188900437764,59.9103237296707));
#21376=CARTESIAN_POINT('Ctrl Pts',(14.6152171518727,-17.3169819821409,59.9540697702187));
#21377=CARTESIAN_POINT('Ctrl Pts',(14.6761902161882,-17.159755202079,59.9768517027666));
#21378=CARTESIAN_POINT('Ctrl Pts',(14.7304276776349,-16.9999999989424,60.0000000001532));
#21379=CARTESIAN_POINT('',(0.,-17.9794361599846,59.8580811200045));
#21380=CARTESIAN_POINT('Origin',(15.75,0.,0.));
#21381=CARTESIAN_POINT('',(15.5,-59.8580811200045,17.9794361599846));
#21382=CARTESIAN_POINT('',(15.4999999969433,-61.0634996055951,13.3228756624643));
#21383=CARTESIAN_POINT('Origin',(15.5,0.,0.));
#21384=CARTESIAN_POINT('Ctrl Pts',(16.,-60.8276253029822,11.9999999999999));
#21385=CARTESIAN_POINT('Ctrl Pts',(16.,-60.8049320488899,12.1150313964023));
#21386=CARTESIAN_POINT('Ctrl Pts',(15.9898935814354,-60.7916707113854,12.2327047392017));
#21387=CARTESIAN_POINT('Ctrl Pts',(15.9261070025809,-60.7835362526876,12.5931700844189));
#21388=CARTESIAN_POINT('Ctrl Pts',(15.8336779042045,-60.8282401952317,12.8299273372328));
#21389=CARTESIAN_POINT('Ctrl Pts',(15.6534629211121,-60.9478909731446,13.1321977587055));
#21390=CARTESIAN_POINT('Ctrl Pts',(15.5800859964154,-61.0013423773347,13.2320666717072));
#21391=CARTESIAN_POINT('Ctrl Pts',(15.4999999966277,-61.0634996097249,13.3228756593561));
#21392=CARTESIAN_POINT('Ctrl Pts',(15.6381526893245,-60.,17.));
#21393=CARTESIAN_POINT('Ctrl Pts',(15.5946215988532,-59.9526427924876,17.3268300981168));
#21394=CARTESIAN_POINT('Ctrl Pts',(15.5485606843564,-59.9053376415117,17.6533009342786));
#21395=CARTESIAN_POINT('Ctrl Pts',(15.5,-59.8580811200045,17.9794361599846));
#21396=CARTESIAN_POINT('Origin',(0.,-59.9290405600022,17.4897180799923));
#21397=CARTESIAN_POINT('',(17.2600442058128,-59.858081116524,17.9794361715722));
#21398=CARTESIAN_POINT('Origin',(18.,-58.,30.8027605631545));
#21399=CARTESIAN_POINT('',(0.,-59.8580811200045,17.9794361599846));
#21400=CARTESIAN_POINT('Origin',(0.,0.,0.));
#21401=CARTESIAN_POINT('',(14.,60.9118215127409,14.));
#21402=CARTESIAN_POINT('Ctrl Pts',(15.499999995189,61.0634996059174,13.3228756609874));
#21403=CARTESIAN_POINT('Ctrl Pts',(15.4701909647076,61.056125041613,13.3566759242301));
#21404=CARTESIAN_POINT('Ctrl Pts',(15.4394885037721,61.0490034120379,13.3891821198367));
#21405=CARTESIAN_POINT('Ctrl Pts',(15.2319678738428,61.0037715519876,13.5949189134652));
#21406=CARTESIAN_POINT('Ctrl Pts',(15.008663619483,60.9694430253741,13.7472835331182));
#21407=CARTESIAN_POINT('Ctrl Pts',(14.5181770858478,60.9234160168088,13.9498447390067));
#21408=CARTESIAN_POINT('Ctrl Pts',(14.2509679895827,60.9118215127409,14.));
#21409=CARTESIAN_POINT('Ctrl Pts',(14.,60.9118215127409,14.));
#21410=CARTESIAN_POINT('',(2.,60.9118215127409,14.));
#21411=CARTESIAN_POINT('',(0.,60.9118215127409,14.));
#21412=CARTESIAN_POINT('',(2.,-60.9118215127409,14.));
#21413=CARTESIAN_POINT('Origin',(2.,0.,0.));
#21414=CARTESIAN_POINT('',(14.,-60.9118215127409,14.));
#21415=CARTESIAN_POINT('',(0.,-60.9118215127409,14.));
#21416=CARTESIAN_POINT('Ctrl Pts',(14.,-60.9118215127409,14.));
#21417=CARTESIAN_POINT('Ctrl Pts',(14.2509679895827,-60.9118215127409,14.));
#21418=CARTESIAN_POINT('Ctrl Pts',(14.5181770858478,-60.9234160168088,13.9498447390067));
#21419=CARTESIAN_POINT('Ctrl Pts',(15.008663619483,-60.9694430253741,13.7472835331182));
#21420=CARTESIAN_POINT('Ctrl Pts',(15.2319678738428,-61.0037715519876,13.5949189134652));
#21421=CARTESIAN_POINT('Ctrl Pts',(15.4394885037721,-61.0490034120379,13.3891821198367));
#21422=CARTESIAN_POINT('Ctrl Pts',(15.4701909647076,-61.056125041613,13.3566759242301));
#21423=CARTESIAN_POINT('Ctrl Pts',(15.499999995189,-61.0634996059174,13.3228756609874));
#21424=CARTESIAN_POINT('',(16.,-58.,23.28626204439));
#21425=CARTESIAN_POINT('Ctrl Pts',(17.2600442115558,-59.8580811153305,17.9794361755454));
#21426=CARTESIAN_POINT('Ctrl Pts',(17.127243690827,-59.8051950958716,18.1555070829828));
#21427=CARTESIAN_POINT('Ctrl Pts',(17.0139600323404,-59.7441024880535,18.3559136759436));
#21428=CARTESIAN_POINT('Ctrl Pts',(16.7810925644696,-59.5935235342901,18.8400023150408));
#21429=CARTESIAN_POINT('Ctrl Pts',(16.6727999393301,-59.5012270640763,19.1293647114412));
#21430=CARTESIAN_POINT('Ctrl Pts',(16.195648993787,-59.0240761185332,20.5909899649672));
#21431=CARTESIAN_POINT('Ctrl Pts',(16.,-58.4904260224498,22.0647388455243));
#21432=CARTESIAN_POINT('Ctrl Pts',(16.,-58.,23.28626204439));
#21433=CARTESIAN_POINT('',(16.,-23.28626204439,58.));
#21434=CARTESIAN_POINT('Origin',(16.,0.,0.));
#21435=CARTESIAN_POINT('Ctrl Pts',(16.,-23.28626204439,58.));
#21436=CARTESIAN_POINT('Ctrl Pts',(16.,-22.0647388455243,58.4904260224498));
#21437=CARTESIAN_POINT('Ctrl Pts',(16.195648993787,-20.5909899649672,59.0240761185332));
#21438=CARTESIAN_POINT('Ctrl Pts',(16.6727999393301,-19.1293647114412,59.5012270640763));
#21439=CARTESIAN_POINT('Ctrl Pts',(16.7810925644696,-18.8400023150408,59.5935235342901));
#21440=CARTESIAN_POINT('Ctrl Pts',(17.0139600323404,-18.3559136759436,59.7441024880535));
#21441=CARTESIAN_POINT('Ctrl Pts',(17.127243690827,-18.1555070829828,59.8051950958716));
#21442=CARTESIAN_POINT('Ctrl Pts',(17.2600442115558,-17.9794361755454,59.8580811153305));
#21443=CARTESIAN_POINT('Origin',(14.,0.,0.));
#21444=CARTESIAN_POINT('',(16.,23.28626204439,58.));
#21445=CARTESIAN_POINT('Ctrl Pts',(17.2600442115558,17.9794361755454,59.8580811153305));
#21446=CARTESIAN_POINT('Ctrl Pts',(17.127243690827,18.1555070829828,59.8051950958716));
#21447=CARTESIAN_POINT('Ctrl Pts',(17.0139600323404,18.3559136759436,59.7441024880535));
#21448=CARTESIAN_POINT('Ctrl Pts',(16.7810925644696,18.8400023150408,59.5935235342901));
#21449=CARTESIAN_POINT('Ctrl Pts',(16.6727999393301,19.1293647114412,59.5012270640763));
#21450=CARTESIAN_POINT('Ctrl Pts',(16.195648993787,20.5909899649672,59.0240761185332));
#21451=CARTESIAN_POINT('Ctrl Pts',(16.,22.0647388455243,58.4904260224498));
#21452=CARTESIAN_POINT('Ctrl Pts',(16.,23.28626204439,58.));
#21453=CARTESIAN_POINT('',(16.,58.,23.28626204439));
#21454=CARTESIAN_POINT('Origin',(16.,0.,0.));
#21455=CARTESIAN_POINT('Ctrl Pts',(16.,58.,23.28626204439));
#21456=CARTESIAN_POINT('Ctrl Pts',(16.,58.4904260224498,22.0647388455243));
#21457=CARTESIAN_POINT('Ctrl Pts',(16.195648993787,59.0240761185332,20.5909899649672));
#21458=CARTESIAN_POINT('Ctrl Pts',(16.6727999393301,59.5012270640763,19.1293647114412));
#21459=CARTESIAN_POINT('Ctrl Pts',(16.7810925644696,59.5935235342901,18.8400023150408));
#21460=CARTESIAN_POINT('Ctrl Pts',(17.0139600323404,59.7441024880535,18.3559136759436));
#21461=CARTESIAN_POINT('Ctrl Pts',(17.127243690827,59.8051950958716,18.1555070829828));
#21462=CARTESIAN_POINT('Ctrl Pts',(17.2600442115558,59.8580811153305,17.9794361755454));
#21463=CARTESIAN_POINT('Origin',(0.25,73.,0.));
#21464=CARTESIAN_POINT('',(0.,73.,7.65));
#21465=CARTESIAN_POINT('Origin',(0.,73.,0.));
#21466=CARTESIAN_POINT('',(0.25,73.,7.4));
#21467=CARTESIAN_POINT('Origin',(0.,0.,0.));
#21468=CARTESIAN_POINT('',(0.,-59.2979763567021,-12.));
#21469=CARTESIAN_POINT('',(0.,59.2979763567021,-12.));
#21470=CARTESIAN_POINT('Origin',(0.,0.,0.));
#21471=CARTESIAN_POINT('',(0.,-73.,-12.));
#21472=CARTESIAN_POINT('',(0.,-36.5,-12.));
#21473=CARTESIAN_POINT('',(0.,-73.,12.));
#21474=CARTESIAN_POINT('Origin',(0.,-73.,0.));
#21475=CARTESIAN_POINT('',(0.,-59.2979763567021,12.));
#21476=CARTESIAN_POINT('',(0.,-30.4559107563704,12.));
#21477=CARTESIAN_POINT('',(0.,59.2979763567021,12.));
#21478=CARTESIAN_POINT('Origin',(0.,0.,0.));
#21479=CARTESIAN_POINT('',(0.,73.,12.));
#21480=CARTESIAN_POINT('',(0.,36.5,12.));
#21481=CARTESIAN_POINT('',(0.,73.,-12.));
#21482=CARTESIAN_POINT('Origin',(0.,73.,0.));
#21483=CARTESIAN_POINT('',(0.,30.4559107563704,-12.));
#21484=CARTESIAN_POINT('',(0.,-73.,7.65));
#21485=CARTESIAN_POINT('Origin',(0.,-73.,0.));
#21486=CARTESIAN_POINT('',(0.,-50.8,-6.22120573966855E-15));
#21487=CARTESIAN_POINT('Origin',(0.,0.,0.));
#21488=CARTESIAN_POINT('Origin',(0.25,-73.,0.));
#21489=CARTESIAN_POINT('',(0.25,-73.,7.4));
#21490=CARTESIAN_POINT('Origin',(2.,0.,0.));
#21491=CARTESIAN_POINT('Ctrl Pts',(0.,59.2979763567021,12.));
#21492=CARTESIAN_POINT('Ctrl Pts',(1.25769149714818E-19,59.2996563019776,
12.0020539660872));
#21493=CARTESIAN_POINT('Ctrl Pts',(3.16408251292899E-6,59.3013362050753,
12.0041079678913));
#21494=CARTESIAN_POINT('Ctrl Pts',(0.000593503086363685,59.4580375808494,
12.1957134154004));
#21495=CARTESIAN_POINT('Ctrl Pts',(0.0281275031880837,59.613099217075,12.3860723403774));
#21496=CARTESIAN_POINT('Ctrl Pts',(0.136930554908868,59.909363508568,12.7511394004012));
#21497=CARTESIAN_POINT('Ctrl Pts',(0.216940282823655,60.0515916827231,12.9270721110806));
#21498=CARTESIAN_POINT('Ctrl Pts',(0.453050831357439,60.3435366239898,13.289351801108));
#21499=CARTESIAN_POINT('Ctrl Pts',(0.62144513700417,60.489695948914,13.4715348257732));
#21500=CARTESIAN_POINT('Ctrl Pts',(0.997206971331434,60.7067257339414,13.7427542799031));
#21501=CARTESIAN_POINT('Ctrl Pts',(1.1889063272169,60.7855458921753,13.8415441416268));
#21502=CARTESIAN_POINT('Ctrl Pts',(1.59182238859041,60.8864806167547,13.9681569376795));
#21503=CARTESIAN_POINT('Ctrl Pts',(1.79387301431878,60.9118215127408,14.));
#21504=CARTESIAN_POINT('Ctrl Pts',(2.,60.9118215127408,14.));
#21505=CARTESIAN_POINT('Ctrl Pts',(0.,-59.2979763567021,12.));
#21506=CARTESIAN_POINT('Ctrl Pts',(1.29042483160331E-19,-59.299700025109,
12.0021074236792));
#21507=CARTESIAN_POINT('Ctrl Pts',(3.33092592262858E-6,-59.3014236491314,
12.0042148849801));
#21508=CARTESIAN_POINT('Ctrl Pts',(0.000607509495687525,-59.4577300699319,
12.1953378269261));
#21509=CARTESIAN_POINT('Ctrl Pts',(0.0280029022425828,-59.6123506019909,
12.3851534403357));
#21510=CARTESIAN_POINT('Ctrl Pts',(0.135984528957224,-59.9071803866406,
12.7484458568845));
#21511=CARTESIAN_POINT('Ctrl Pts',(0.215085926484061,-60.0484388333809,
12.9231705561954));
#21512=CARTESIAN_POINT('Ctrl Pts',(0.449932961616034,-60.3406955295315,
13.2858134156949));
#21513=CARTESIAN_POINT('Ctrl Pts',(0.618802310815173,-60.4878960201855,
13.4692879696251));
#21514=CARTESIAN_POINT('Ctrl Pts',(0.995804745415966,-60.7061337709478,
13.7420125229231));
#21515=CARTESIAN_POINT('Ctrl Pts',(1.18797810444438,-60.7852814744256,13.8412125450258));
#21516=CARTESIAN_POINT('Ctrl Pts',(1.59159091693634,-60.8864513713538,13.9681201712759));
#21517=CARTESIAN_POINT('Ctrl Pts',(1.79375386609647,-60.9118215127408,14.));
#21518=CARTESIAN_POINT('Ctrl Pts',(2.,-60.9118215127408,14.));
#21519=CARTESIAN_POINT('Origin',(2.,-30.4559107563704,12.));
#21520=CARTESIAN_POINT('',(2.,-73.,14.));
#21521=CARTESIAN_POINT('Origin',(2.,-73.,12.));
#21522=CARTESIAN_POINT('',(2.,-30.4559107563704,14.));
#21523=CARTESIAN_POINT('Origin',(2.,-73.,0.));
#21524=CARTESIAN_POINT('',(2.,-73.,-14.));
#21525=CARTESIAN_POINT('Origin',(2.,-73.,-12.));
#21526=CARTESIAN_POINT('Origin',(2.,-73.,0.));
#21527=CARTESIAN_POINT('Origin',(2.,-36.5,-12.));
#21528=CARTESIAN_POINT('Ctrl Pts',(2.,-60.9118215127409,-14.));
#21529=CARTESIAN_POINT('Ctrl Pts',(1.79662005343113,-60.9118215127409,-14.));
#21530=CARTESIAN_POINT('Ctrl Pts',(1.59716111634269,-60.8871502501852,-13.9689987706081));
#21531=CARTESIAN_POINT('Ctrl Pts',(1.20761476381752,-60.7909127959859,-13.8482745236258));
#21532=CARTESIAN_POINT('Ctrl Pts',(1.02476537018483,-60.7182038738797,-13.7571370843373));
#21533=CARTESIAN_POINT('Ctrl Pts',(0.667985559569145,-60.5210049472671,
-13.5106227806572));
#21534=CARTESIAN_POINT('Ctrl Pts',(0.506200805332197,-60.3904050016375,
-13.347738482477));
#21535=CARTESIAN_POINT('Ctrl Pts',(0.249110343832778,-60.10362247768,-12.9914917064196));
#21536=CARTESIAN_POINT('Ctrl Pts',(0.154074961880266,-59.9469693395654,
-12.7975571845823));
#21537=CARTESIAN_POINT('Ctrl Pts',(0.0308705553692023,-59.6282594152053,
-12.4046866976145));
#21538=CARTESIAN_POINT('Ctrl Pts',(0.0006041682808588,-59.465531757485,
-12.2048763799246));
#21539=CARTESIAN_POINT('Ctrl Pts',(2.98520635993023E-6,-59.3012398529037,
-12.0039901590642));
#21540=CARTESIAN_POINT('Ctrl Pts',(-8.73769579204139E-18,-59.2996081247075,
-12.0019950626929));
#21541=CARTESIAN_POINT('Ctrl Pts',(0.,-59.2979763567021,-12.));
#21542=CARTESIAN_POINT('',(2.,-36.5,-14.));
#21543=CARTESIAN_POINT('Origin',(2.,0.,0.));
#21544=CARTESIAN_POINT('Ctrl Pts',(0.,59.2979763567021,-12.));
#21545=CARTESIAN_POINT('Ctrl Pts',(-9.22979868187932E-18,59.299700025109,
-12.0021074236792));
#21546=CARTESIAN_POINT('Ctrl Pts',(3.3309259227759E-6,59.3014236491314,
-12.0042148849801));
#21547=CARTESIAN_POINT('Ctrl Pts',(0.000607509495675756,59.4577300699289,
-12.1953378269221));
#21548=CARTESIAN_POINT('Ctrl Pts',(0.0280029022423892,59.6123506019904,
-12.385153440335));
#21549=CARTESIAN_POINT('Ctrl Pts',(0.135984528957217,59.9071803866406,-12.7484458568844));
#21550=CARTESIAN_POINT('Ctrl Pts',(0.215085926484053,60.0484388333809,-12.9231705561954));
#21551=CARTESIAN_POINT('Ctrl Pts',(0.449932961616014,60.3406955295314,-13.2858134156948));
#21552=CARTESIAN_POINT('Ctrl Pts',(0.618802310815157,60.4878960201855,-13.4692879696251));
#21553=CARTESIAN_POINT('Ctrl Pts',(0.995804745415989,60.7061337709478,-13.7420125229231));
#21554=CARTESIAN_POINT('Ctrl Pts',(1.18797810444439,60.7852814744256,-13.8412125450258));
#21555=CARTESIAN_POINT('Ctrl Pts',(1.59159091693627,60.8864513713538,-13.9681201712759));
#21556=CARTESIAN_POINT('Ctrl Pts',(1.79375386609643,60.9118215127409,-14.));
#21557=CARTESIAN_POINT('Ctrl Pts',(2.,60.9118215127409,-14.));
#21558=CARTESIAN_POINT('Origin',(2.,73.,0.));
#21559=CARTESIAN_POINT('',(2.,73.,-14.));
#21560=CARTESIAN_POINT('Origin',(2.,73.,-12.));
#21561=CARTESIAN_POINT('',(2.,73.,14.));
#21562=CARTESIAN_POINT('Origin',(2.,73.,12.));
#21563=CARTESIAN_POINT('Origin',(2.,73.,0.));
#21564=CARTESIAN_POINT('Origin',(2.,36.5,12.));
#21565=CARTESIAN_POINT('',(2.,36.5,14.));
#21566=CARTESIAN_POINT('Origin',(2.,30.4559107563704,-12.));
#21567=CARTESIAN_POINT('',(2.,30.4559107563704,-14.));
#21568=CARTESIAN_POINT('Origin',(0.,73.,0.));
#21569=CARTESIAN_POINT('',(14.,73.,14.));
#21570=CARTESIAN_POINT('',(0.,73.,14.));
#21571=CARTESIAN_POINT('',(14.,73.,-14.));
#21572=CARTESIAN_POINT('Origin',(14.,73.,0.));
#21573=CARTESIAN_POINT('',(0.,73.,-14.));
#21574=CARTESIAN_POINT('Origin',(0.,73.,14.));
#21575=CARTESIAN_POINT('',(14.,36.5,14.));
#21576=CARTESIAN_POINT('Origin',(14.,0.,0.));
#21577=CARTESIAN_POINT('Origin',(16.,0.,0.));
#21578=CARTESIAN_POINT('Origin',(14.,-30.4559107563704,12.));
#21579=CARTESIAN_POINT('',(14.,-73.,14.));
#21580=CARTESIAN_POINT('Origin',(14.,-73.,12.));
#21581=CARTESIAN_POINT('',(14.,-30.4559107563704,14.));
#21582=CARTESIAN_POINT('Origin',(14.,-73.,0.));
#21583=CARTESIAN_POINT('',(14.,-73.,-14.));
#21584=CARTESIAN_POINT('Origin',(14.,-73.,-12.));
#21585=CARTESIAN_POINT('Origin',(14.,-73.,0.));
#21586=CARTESIAN_POINT('Origin',(14.,-36.5,-12.));
#21587=CARTESIAN_POINT('',(14.,-36.5,-14.));
#21588=CARTESIAN_POINT('Origin',(0.,-73.,-14.));
#21589=CARTESIAN_POINT('',(0.,-73.,-14.));
#21590=CARTESIAN_POINT('Origin',(0.,-73.,0.));
#21591=CARTESIAN_POINT('',(0.,-73.,14.));
#21592=CARTESIAN_POINT('Origin',(0.,-60.9118215127409,14.));
#21593=CARTESIAN_POINT('Origin',(14.,0.,0.));
#21594=CARTESIAN_POINT('Origin',(16.,0.,0.));
#21595=CARTESIAN_POINT('Origin',(14.,30.4559107563704,-12.));
#21596=CARTESIAN_POINT('Origin',(14.,73.,-12.));
#21597=CARTESIAN_POINT('',(14.,30.4559107563704,-14.));
#21598=CARTESIAN_POINT('Origin',(14.,73.,0.));
#21599=CARTESIAN_POINT('Origin',(14.,73.,12.));
#21600=CARTESIAN_POINT('Origin',(14.,36.5,12.));
#21601=CARTESIAN_POINT('Origin',(0.,60.9118215127409,-14.));
#21602=CARTESIAN_POINT('Origin',(-8.17712434446771,0.,0.));
#21603=CARTESIAN_POINT('',(-8.17712434446771,-50.8,1.55887483312148E-14));
#21604=CARTESIAN_POINT('Origin',(-8.17712434446771,0.,0.));
#21605=CARTESIAN_POINT('',(-9.5,-50.3,1.54353157688997E-14));
#21606=CARTESIAN_POINT('Origin',(-8.17712434446771,-48.8,1.49750180819544E-14));
#21607=CARTESIAN_POINT('Origin',(-9.5,0.,0.));
#21608=CARTESIAN_POINT('Origin',(-4.45,0.,0.));
#21609=CARTESIAN_POINT('',(-4.45,-50.8,-6.22120573966855E-15));
#21610=CARTESIAN_POINT('Origin',(18.,16.,58.));
#21611=CARTESIAN_POINT('',(16.,-32.,58.));
#21612=CARTESIAN_POINT('',(16.,16.,58.));
#21613=CARTESIAN_POINT('Origin',(18.,-32.,58.));
#21614=CARTESIAN_POINT('Origin',(18.,-32.,32.));
#21615=CARTESIAN_POINT('',(16.,-58.,32.));
#21616=CARTESIAN_POINT('Origin',(18.,-58.,32.));
#21617=CARTESIAN_POINT('Origin',(18.,-32.,32.));
#21618=CARTESIAN_POINT('Origin',(16.,-32.,32.));
#21619=CARTESIAN_POINT('Origin',(18.,-58.,16.));
#21620=CARTESIAN_POINT('',(16.,-58.,16.));
#21621=CARTESIAN_POINT('Origin',(16.,0.,0.));
#21622=CARTESIAN_POINT('Origin',(18.,32.,32.));
#21623=CARTESIAN_POINT('',(16.,58.,32.));
#21624=CARTESIAN_POINT('Origin',(18.,58.,32.));
#21625=CARTESIAN_POINT('',(16.,32.,58.));
#21626=CARTESIAN_POINT('Origin',(16.,32.,32.));
#21627=CARTESIAN_POINT('Origin',(18.,32.,58.));
#21628=CARTESIAN_POINT('Origin',(18.,32.,32.));
#21629=CARTESIAN_POINT('Origin',(18.,16.,58.));
#21630=CARTESIAN_POINT('',(16.,16.,58.));
#21631=CARTESIAN_POINT('Origin',(18.,58.,-16.));
#21632=CARTESIAN_POINT('',(16.,58.,-16.));
#21633=CARTESIAN_POINT('Origin',(16.,0.,0.));
#21634=CARTESIAN_POINT('Origin',(18.,-16.,-58.));
#21635=CARTESIAN_POINT('',(16.,32.,-58.));
#21636=CARTESIAN_POINT('',(16.,-16.,-58.));
#21637=CARTESIAN_POINT('Origin',(18.,32.,-58.));
#21638=CARTESIAN_POINT('Origin',(18.,32.,-32.));
#21639=CARTESIAN_POINT('',(16.,58.,-32.));
#21640=CARTESIAN_POINT('Origin',(18.,58.,-32.));
#21641=CARTESIAN_POINT('Origin',(18.,32.,-32.));
#21642=CARTESIAN_POINT('Origin',(16.,32.,-32.));
#21643=CARTESIAN_POINT('Origin',(18.,58.,-16.));
#21644=CARTESIAN_POINT('',(16.,58.,-16.));
#21645=CARTESIAN_POINT('Origin',(16.,0.,0.));
#21646=CARTESIAN_POINT('Origin',(18.,-58.,16.));
#21647=CARTESIAN_POINT('',(16.,-58.,-32.));
#21648=CARTESIAN_POINT('',(16.,-58.,16.));
#21649=CARTESIAN_POINT('Origin',(18.,-58.,-32.));
#21650=CARTESIAN_POINT('Origin',(18.,-32.,-32.));
#21651=CARTESIAN_POINT('',(16.,-32.,-58.));
#21652=CARTESIAN_POINT('Origin',(18.,-32.,-58.));
#21653=CARTESIAN_POINT('Origin',(18.,-32.,-32.));
#21654=CARTESIAN_POINT('Origin',(16.,-32.,-32.));
#21655=CARTESIAN_POINT('Origin',(18.,-16.,-58.));
#21656=CARTESIAN_POINT('',(16.,-16.,-58.));
#21657=CARTESIAN_POINT('Origin',(16.,0.,0.));
#21658=CARTESIAN_POINT('Origin',(123.8,-16.,-58.));
#21659=CARTESIAN_POINT('Origin',(123.8,-32.,-58.));
#21660=CARTESIAN_POINT('Origin',(123.8,32.,-58.));
#21661=CARTESIAN_POINT('Origin',(123.8,32.,-32.));
#21662=CARTESIAN_POINT('Origin',(123.8,58.,-32.));
#21663=CARTESIAN_POINT('Origin',(123.8,32.,-32.));
#21664=CARTESIAN_POINT('Origin',(123.8,58.,-16.));
#21665=CARTESIAN_POINT('Origin',(123.8,58.,32.));
#21666=CARTESIAN_POINT('Origin',(123.8,32.,32.));
#21667=CARTESIAN_POINT('Origin',(123.8,32.,58.));
#21668=CARTESIAN_POINT('Origin',(123.8,32.,32.));
#21669=CARTESIAN_POINT('Origin',(123.8,16.,58.));
#21670=CARTESIAN_POINT('Origin',(123.8,-32.,58.));
#21671=CARTESIAN_POINT('Origin',(123.8,-32.,32.));
#21672=CARTESIAN_POINT('Origin',(123.8,-58.,32.));
#21673=CARTESIAN_POINT('Origin',(123.8,-32.,32.));
#21674=CARTESIAN_POINT('Origin',(123.8,-58.,16.));
#21675=CARTESIAN_POINT('Origin',(123.8,-58.,-32.));
#21676=CARTESIAN_POINT('Origin',(123.8,-32.,-32.));
#21677=CARTESIAN_POINT('Origin',(123.8,-32.,-32.));
#21678=CARTESIAN_POINT('Origin',(16.,32.,32.));
#21679=CARTESIAN_POINT('Origin',(16.,32.,-32.));
#21680=CARTESIAN_POINT('Origin',(123.8,0.,0.));
#21681=CARTESIAN_POINT('',(123.8,-6.12323399573677E-15,-50.));
#21682=CARTESIAN_POINT('Origin',(123.8,-6.36816335556624E-15,-52.));
#21683=CARTESIAN_POINT('',(123.8,-50.,6.12323399573677E-15));
#21684=CARTESIAN_POINT('Origin',(123.8,0.,0.));
#21685=CARTESIAN_POINT('Origin',(123.8,0.,0.));
#21686=CARTESIAN_POINT('Origin',(70.95,0.,0.));
#21687=CARTESIAN_POINT('',(16.,-50.,-6.12323399573677E-15));
#21688=CARTESIAN_POINT('Origin',(16.,0.,0.));
#21689=CARTESIAN_POINT('',(70.95,-50.,-6.12323399573677E-15));
#21690=CARTESIAN_POINT('',(71.6135123314049,23.3160685634306,44.2307692307674));
#21691=CARTESIAN_POINT('',(73.2907028363675,19.5959875136913,46.0001627885347));
#21692=CARTESIAN_POINT('Ctrl Pts',(71.6135123314072,23.3160685634275,44.2307692307691));
#21693=CARTESIAN_POINT('Ctrl Pts',(71.6932714543115,23.2042169236777,44.2897313638428));
#21694=CARTESIAN_POINT('Ctrl Pts',(71.8483990288815,22.9774859633438,44.4081667977607));
#21695=CARTESIAN_POINT('Ctrl Pts',(72.0309897669014,22.6869514584429,44.557072726346));
#21696=CARTESIAN_POINT('Ctrl Pts',(72.1700773346563,22.4505358369901,44.6764670164254));
#21697=CARTESIAN_POINT('Ctrl Pts',(72.3044475744177,22.211560601306,44.7959596617311));
#21698=CARTESIAN_POINT('Ctrl Pts',(72.4157517404387,21.9992281010938,44.9005387053819));
#21699=CARTESIAN_POINT('Ctrl Pts',(72.5065732598677,21.8151167092688,44.990045399374));
#21700=CARTESIAN_POINT('Ctrl Pts',(72.5658930280084,21.6918256295662,45.0496717620424));
#21701=CARTESIAN_POINT('Ctrl Pts',(72.6377280503905,21.5367060266982,45.1241021330032));
#21702=CARTESIAN_POINT('Ctrl Pts',(72.7201916785671,21.3490306679124,45.2131989345674));
#21703=CARTESIAN_POINT('Ctrl Pts',(72.7988814082159,21.1599111909158,45.302017540834));
#21704=CARTESIAN_POINT('Ctrl Pts',(72.8737703412485,20.969415619956,45.3905097941917));
#21705=CARTESIAN_POINT('Ctrl Pts',(72.9448178995343,20.7776647362872,45.4786056970811));
#21706=CARTESIAN_POINT('Ctrl Pts',(73.0121109467716,20.5844107113345,45.5664035981079));
#21707=CARTESIAN_POINT('Ctrl Pts',(73.0755852718533,20.3897951762557,45.6538223879631));
#21708=CARTESIAN_POINT('Ctrl Pts',(73.1352131070871,20.1938738237251,45.7408225076835));
#21709=CARTESIAN_POINT('Ctrl Pts',(73.1909498335265,19.9967609507555,45.8273396719058));
#21710=CARTESIAN_POINT('Ctrl Pts',(73.2341485984696,19.8314987172849,45.8990281581236));
#21711=CARTESIAN_POINT('Ctrl Pts',(73.2626675329748,19.7153221034526,45.9489756536103));
#21712=CARTESIAN_POINT('Ctrl Pts',(73.278471643703,19.6487953456216,45.977449084781));
#21713=CARTESIAN_POINT('Ctrl Pts',(73.2862090342068,19.6154867193585,45.9916623858903));
#21714=CARTESIAN_POINT('Ctrl Pts',(73.2902585153488,19.5978545384253,45.9991749778942));
#21715=CARTESIAN_POINT('Ctrl Pts',(73.2904803873088,19.5968878248965,45.9995868316516));
#21716=CARTESIAN_POINT('Ctrl Pts',(73.2907028377334,19.5959211154461,45.9999986482306));
#21717=CARTESIAN_POINT('',(53.3864876668068,23.3160685609229,44.2307692320894));
#21718=CARTESIAN_POINT('Ctrl Pts',(53.3864876668068,23.3160685609229,44.2307692320894));
#21719=CARTESIAN_POINT('Ctrl Pts',(53.8964899676441,24.0312794561666,43.8537487425402));
#21720=CARTESIAN_POINT('Ctrl Pts',(55.3186828044349,25.2435158958716,43.1695330127632));
#21721=CARTESIAN_POINT('Ctrl Pts',(58.0747486677894,26.2360703120526,42.564673612103));
#21722=CARTESIAN_POINT('Ctrl Pts',(61.020309894555,26.5481066493621,42.3696710366589));
#21723=CARTESIAN_POINT('Ctrl Pts',(63.9663874943631,26.5460492373018,42.3707472230138));
#21724=CARTESIAN_POINT('Ctrl Pts',(66.9244886027247,26.2356604580669,42.5652091566662));
#21725=CARTESIAN_POINT('Ctrl Pts',(69.681226557465,25.239555364586,43.1717497595138));
#21726=CARTESIAN_POINT('Ctrl Pts',(71.0985268893462,24.038267655457,43.8500649418989));
#21727=CARTESIAN_POINT('Ctrl Pts',(71.6135123314272,23.3160685633993,44.2307692307839));
#21728=CARTESIAN_POINT('',(51.7092971474407,19.5959037569241,45.9999667943664));
#21729=CARTESIAN_POINT('Ctrl Pts',(51.7092971610549,19.5959179422654,46.));
#21730=CARTESIAN_POINT('Ctrl Pts',(51.7312389779497,19.6914330268016,45.959302575355));
#21731=CARTESIAN_POINT('Ctrl Pts',(51.8239020992648,20.0709136872745,45.7962695577249));
#21732=CARTESIAN_POINT('Ctrl Pts',(52.0530341102106,20.8197959816443,45.4633470605684));
#21733=CARTESIAN_POINT('Ctrl Pts',(52.5423502486883,21.9908524941898,44.9125177602508));
#21734=CARTESIAN_POINT('Ctrl Pts',(53.0439951189989,22.8358340303902,44.4839588612342));
#21735=CARTESIAN_POINT('Ctrl Pts',(53.3864876668068,23.3160685609229,44.2307692320894));
#21736=CARTESIAN_POINT('Ctrl Pts',(73.2907028363675,19.5959875136913,46.0001627885347));
#21737=CARTESIAN_POINT('Ctrl Pts',(73.3614481346313,19.2876918400925,46.1319200512155));
#21738=CARTESIAN_POINT('Ctrl Pts',(73.4180753927526,18.9755505935139,46.2617120261331));
#21739=CARTESIAN_POINT('Ctrl Pts',(73.4601341604197,18.6605239219579,46.3888396110071));
#21740=CARTESIAN_POINT('Ctrl Pts',(73.4994000293548,18.3664164936491,46.5075253301233));
#21741=CARTESIAN_POINT('Ctrl Pts',(73.5260008275866,18.0698024364483,46.6238849103412));
#21742=CARTESIAN_POINT('Ctrl Pts',(73.5395273739608,17.7715244162219,46.737334373478));
#21743=CARTESIAN_POINT('Ctrl Pts',(73.5451949896521,17.6465460853884,46.784869637813));
#21744=CARTESIAN_POINT('Ctrl Pts',(73.5485678818421,17.521275662251,46.8318941375462));
#21745=CARTESIAN_POINT('Ctrl Pts',(73.5496186134852,17.395775144484,46.8783656049086));
#21746=CARTESIAN_POINT('Ctrl Pts',(73.550638568793,17.273950585317,46.9234759050572));
#21747=CARTESIAN_POINT('Ctrl Pts',(73.549470420523,17.1519092272119,46.9680651041026));
#21748=CARTESIAN_POINT('Ctrl Pts',(73.546122975365,17.0297456445921,47.0121211853996));
#21749=CARTESIAN_POINT('Ctrl Pts',(73.5385114955969,16.7519679384259,47.1122966791343));
#21750=CARTESIAN_POINT('Ctrl Pts',(73.5190626012108,16.473522026003,47.2097294454252));
#21751=CARTESIAN_POINT('Ctrl Pts',(73.488046964858,16.1953398787474,47.3043376488432));
#21752=CARTESIAN_POINT('Ctrl Pts',(73.4591781610324,15.9364128734918,47.3923972853989));
#21753=CARTESIAN_POINT('Ctrl Pts',(73.420288919625,15.6777138858939,47.4780101963045));
#21754=CARTESIAN_POINT('Ctrl Pts',(73.3715757825718,15.4199486044262,47.5611191306938));
#21755=CARTESIAN_POINT('Ctrl Pts',(73.3679532235023,15.4007798541739,47.5672995379154));
#21756=CARTESIAN_POINT('Ctrl Pts',(73.3642763241121,15.3816162471717,47.5734661006511));
#21757=CARTESIAN_POINT('Ctrl Pts',(73.3605451589308,15.3624580638881,47.5796187966842));
#21758=CARTESIAN_POINT('Ctrl Pts',(73.3071301487798,15.0881913121253,47.6677002149798));
#21759=CARTESIAN_POINT('Ctrl Pts',(73.2425888013964,14.8149979710872,47.7529521629476));
#21760=CARTESIAN_POINT('Ctrl Pts',(73.1668141764284,14.5438139588109,47.8352695279082));
#21761=CARTESIAN_POINT('Ctrl Pts',(73.0918525519906,14.2755395319778,47.9167036940224));
#21762=CARTESIAN_POINT('Ctrl Pts',(73.0058967816236,14.0092312159786,47.9952657482102));
#21763=CARTESIAN_POINT('Ctrl Pts',(72.9088264267727,13.7458407566761,48.0708394050032));
#21764=CARTESIAN_POINT('Ctrl Pts',(72.8316347408528,13.536389028185,48.130936619935));
#21765=CARTESIAN_POINT('Ctrl Pts',(72.7474141369172,13.3287833016545,48.1891437526931));
#21766=CARTESIAN_POINT('Ctrl Pts',(72.6561002844086,13.1235248126055,48.2453968530772));
#21767=CARTESIAN_POINT('Ctrl Pts',(72.5316712735188,12.8438289059336,48.3220502572211));
#21768=CARTESIAN_POINT('Ctrl Pts',(72.3946427652386,12.5682553157748,48.3951379950373));
#21769=CARTESIAN_POINT('Ctrl Pts',(72.245053609984,12.2981649671315,48.464464920355));
#21770=CARTESIAN_POINT('Ctrl Pts',(72.0983246196883,12.0332387826257,48.5324663054478));
#21771=CARTESIAN_POINT('Ctrl Pts',(71.939510779376,11.7735888662279,48.5968492518765));
#21772=CARTESIAN_POINT('Ctrl Pts',(71.7686966780188,11.5204923924152,48.6574411642038));
#21773=CARTESIAN_POINT('Ctrl Pts',(71.7001573486202,11.4189371785865,48.6817537297643));
#21774=CARTESIAN_POINT('Ctrl Pts',(71.6296864904025,11.3184369448846,48.705456067353));
#21775=CARTESIAN_POINT('Ctrl Pts',(71.5572917659591,11.2190734726146,48.7285376036628));
#21776=CARTESIAN_POINT('Ctrl Pts',(71.3768963941771,10.9714765564093,48.786052876439));
#21777=CARTESIAN_POINT('Ctrl Pts',(71.184552308396,10.7309398968218,48.8397126227416));
#21778=CARTESIAN_POINT('Ctrl Pts',(70.9813698482786,10.4983816308439,48.8897537967881));
#21779=CARTESIAN_POINT('Ctrl Pts',(70.7778012863261,10.2653814410245,48.9398900626508));
#21780=CARTESIAN_POINT('Ctrl Pts',(70.5633536284789,10.0403906456116,48.9863940944043));
#21781=CARTESIAN_POINT('Ctrl Pts',(70.3391832313088,9.8243010871711,49.0295155385523));
#21782=CARTESIAN_POINT('Ctrl Pts',(70.3154954232116,9.80146717128941,49.0340721281232));
#21783=CARTESIAN_POINT('Ctrl Pts',(70.2916990842856,9.77873261128666,49.0385909576319));
#21784=CARTESIAN_POINT('Ctrl Pts',(70.2677956009778,9.75609843423282,49.043072328228));
#21785=CARTESIAN_POINT('Ctrl Pts',(70.0118710660855,9.51376382715578,49.0910524770088));
#21786=CARTESIAN_POINT('Ctrl Pts',(69.7432342365535,9.28302248963847,49.1347219741822));
#21787=CARTESIAN_POINT('Ctrl Pts',(69.463336662313,9.06493981195789,49.1744863022742));
#21788=CARTESIAN_POINT('Ctrl Pts',(69.18146262429,8.84531716911266,49.2145314214896));
#21789=CARTESIAN_POINT('Ctrl Pts',(68.8881677361653,8.63853183864154,49.2506159507198));
#21790=CARTESIAN_POINT('Ctrl Pts',(68.5848877717148,8.44569449976274,49.2831415609367));
#21791=CARTESIAN_POINT('Ctrl Pts',(68.2845080196753,8.2547012300909,49.3153561345226));
#21792=CARTESIAN_POINT('Ctrl Pts',(67.9743325950966,8.07738978136323,49.3440794037022));
#21793=CARTESIAN_POINT('Ctrl Pts',(67.6557196810578,7.91487194608282,49.3696909984755));
#21794=CARTESIAN_POINT('Ctrl Pts',(67.3613870476161,7.76473897804652,49.3933508308431));
#21795=CARTESIAN_POINT('Ctrl Pts',(67.0598531374047,7.62723068755149,49.414354985105));
#21796=CARTESIAN_POINT('Ctrl Pts',(66.7521676869351,7.50325643845802,49.4329960508709));
#21797=CARTESIAN_POINT('Ctrl Pts',(66.50225675491,7.40256100391349,49.448136858187));
#21798=CARTESIAN_POINT('Ctrl Pts',(66.2484614297923,7.31061703715261,49.4617452712725));
#21799=CARTESIAN_POINT('Ctrl Pts',(65.9913615551387,7.2279790305136,49.4739653333684));
#21800=CARTESIAN_POINT('Ctrl Pts',(65.6570871797071,7.12053530618906,49.4898535310205));
#21801=CARTESIAN_POINT('Ctrl Pts',(65.3172247744756,7.02882321195569,49.5033947318101));
#21802=CARTESIAN_POINT('Ctrl Pts',(64.9734117791745,6.95299333693358,49.5145694818844));
#21803=CARTESIAN_POINT('Ctrl Pts',(64.6278849499738,6.87678546627959,49.5257999356865));
#21804=CARTESIAN_POINT('Ctrl Pts',(64.2783681408376,6.81661934572417,49.5346403474515));
#21805=CARTESIAN_POINT('Ctrl Pts',(63.9265760227067,6.7726460431142,49.5410742954058));
#21806=CARTESIAN_POINT('Ctrl Pts',(63.5742519227226,6.72860624384951,49.5475179728092));
#21807=CARTESIAN_POINT('Ctrl Pts',(63.2196458701498,6.70080908424267,49.5515479323014));
#21808=CARTESIAN_POINT('Ctrl Pts',(62.8645303999073,6.68939242925534,49.5531503258018));
#21809=CARTESIAN_POINT('Ctrl Pts',(62.7430551295141,6.6854871044588,49.5536984607045));
#21810=CARTESIAN_POINT('Ctrl Pts',(62.6215206631554,6.68349834754966,49.5539625582977));
#21811=CARTESIAN_POINT('Ctrl Pts',(62.499999199999,6.6834310420419,49.5539421295715));
#21812=CARTESIAN_POINT('Ctrl Pts',(62.1897600464977,6.68325921392849,49.553889975898));
#21813=CARTESIAN_POINT('Ctrl Pts',(61.8794936145935,6.69574259278768,49.5519656432217));
#21814=CARTESIAN_POINT('Ctrl Pts',(61.5703573069878,6.7207420019746,49.5481895211902));
#21815=CARTESIAN_POINT('Ctrl Pts',(61.2608873346803,6.74576839414671,49.5444093234207));
#21816=CARTESIAN_POINT('Ctrl Pts',(60.9525498130144,6.78333706171612,49.5387733420942));
#21817=CARTESIAN_POINT('Ctrl Pts',(60.6464542896073,6.83331469294025,49.5313004859268));
#21818=CARTESIAN_POINT('Ctrl Pts',(60.523559121281,6.85338035523245,49.5283001875025));
#21819=CARTESIAN_POINT('Ctrl Pts',(60.4010247844408,6.87544643607457,49.5250037737621));
#21820=CARTESIAN_POINT('Ctrl Pts',(60.2789208350937,6.89950503634368,49.5214124066634));
#21821=CARTESIAN_POINT('Ctrl Pts',(59.9277856936677,6.96869051357988,49.5110846883473));
#21822=CARTESIAN_POINT('Ctrl Pts',(59.5801503156904,7.05408058719238,49.4983547685931));
#21823=CARTESIAN_POINT('Ctrl Pts',(59.2378514600242,7.15571464542734,49.4832256563387));
#21824=CARTESIAN_POINT('Ctrl Pts',(59.1609163729305,7.1785579152559,49.4798252372322));
#21825=CARTESIAN_POINT('Ctrl Pts',(59.0842508602296,7.20222158226451,49.4763036692557));
#21826=CARTESIAN_POINT('Ctrl Pts',(59.0078757360508,7.22670573976275,49.4726610750435));
#21827=CARTESIAN_POINT('Ctrl Pts',(58.6908785430507,7.32832795358386,49.4575423809281));
#21828=CARTESIAN_POINT('Ctrl Pts',(58.3788847972949,7.44408741355368,49.4403379670896));
#21829=CARTESIAN_POINT('Ctrl Pts',(58.0730988777378,7.5729945695746,49.4207696740327));
#21830=CARTESIAN_POINT('Ctrl Pts',(57.74966674389,7.70934066621787,49.4000721390112));
#21831=CARTESIAN_POINT('Ctrl Pts',(57.4334521150688,7.8608904174952,49.3766553872395));
#21832=CARTESIAN_POINT('Ctrl Pts',(57.1256864306589,8.02646056782285,49.3501805334311));
#21833=CARTESIAN_POINT('Ctrl Pts',(56.814041913381,8.19411743208113,49.3233720117114));
#21834=CARTESIAN_POINT('Ctrl Pts',(56.5110598816884,8.37615053289667,49.2934279876878));
#21835=CARTESIAN_POINT('Ctrl Pts',(56.218019637168,8.57138477273958,49.2599889073673));
#21836=CARTESIAN_POINT('Ctrl Pts',(55.9242821674943,8.76708352974473,49.2264702660706));
#21837=CARTESIAN_POINT('Ctrl Pts',(55.6405329777448,8.9760466670762,49.1894401167517));
#21838=CARTESIAN_POINT('Ctrl Pts',(55.3680736173629,9.19713973768636,49.148525887908));
#21839=CARTESIAN_POINT('Ctrl Pts',(55.2153011969308,9.32111023916053,49.1255846104939));
#21840=CARTESIAN_POINT('Ctrl Pts',(55.0660786369272,9.44889527856915,49.1014219643564));
#21841=CARTESIAN_POINT('Ctrl Pts',(54.9206388099483,9.58030092990195,49.0759704510606));
#21842=CARTESIAN_POINT('Ctrl Pts',(54.6873329934736,9.79109396651661,49.0351426653478));
#21843=CARTESIAN_POINT('Ctrl Pts',(54.4635724344831,10.0113464810153,48.9909702843494));
#21844=CARTESIAN_POINT('Ctrl Pts',(54.2505163116649,10.2400992217127,48.9431994614762));
#21845=CARTESIAN_POINT('Ctrl Pts',(54.0371783773243,10.4691545360102,48.8953654516448));
#21846=CARTESIAN_POINT('Ctrl Pts',(53.8345735518,10.7067318313352,48.8439234119285));
#21847=CARTESIAN_POINT('Ctrl Pts',(53.6438198607322,10.9518453411613,48.7886281792624));
#21848=CARTESIAN_POINT('Ctrl Pts',(53.5751826699505,11.0400423382571,48.7687317913468));
#21849=CARTESIAN_POINT('Ctrl Pts',(53.5080794064406,11.1292148992273,48.7483366211777));
#21850=CARTESIAN_POINT('Ctrl Pts',(53.4425605926292,11.2193166643701,48.7274315729019));
#21851=CARTESIAN_POINT('Ctrl Pts',(53.2598511346751,11.4705795263217,48.6691345767143));
#21852=CARTESIAN_POINT('Ctrl Pts',(53.0894670854084,11.7290686403632,48.6068717193985));
#21853=CARTESIAN_POINT('Ctrl Pts',(52.9314780004343,11.9934610506509,48.5408180490906));
#21854=CARTESIAN_POINT('Ctrl Pts',(52.7697206955817,12.2641595214891,48.4731889234052));
#21855=CARTESIAN_POINT('Ctrl Pts',(52.6209565156028,12.5410454414813,48.4015861388442));
#21856=CARTESIAN_POINT('Ctrl Pts',(52.4852071420199,12.8227024785657,48.3262070143474));
#21857=CARTESIAN_POINT('Ctrl Pts',(52.4676741301488,12.8590805188059,48.3164712560913));
#21858=CARTESIAN_POINT('Ctrl Pts',(52.4503581571292,12.8955381632686,48.3066725134332));
#21859=CARTESIAN_POINT('Ctrl Pts',(52.4332592094338,12.9320723751521,48.2968112208205));
#21860=CARTESIAN_POINT('Ctrl Pts',(52.3034526058899,13.2094217209856,48.221949251335));
#21861=CARTESIAN_POINT('Ctrl Pts',(52.1866217579404,13.4913117239867,48.1434486683242));
#21862=CARTESIAN_POINT('Ctrl Pts',(52.0826632708201,13.7765258626941,48.0614627034639));
#21863=CARTESIAN_POINT('Ctrl Pts',(51.9773786777555,14.0653782244576,47.9784309165802));
#21864=CARTESIAN_POINT('Ctrl Pts',(51.8852963255834,14.3576403533906,47.891824431865));
#21865=CARTESIAN_POINT('Ctrl Pts',(51.8063250046279,14.6520979265174,47.8017885914336));
#21866=CARTESIAN_POINT('Ctrl Pts',(51.7541270394914,14.8467266341326,47.7422772700703));
#21867=CARTESIAN_POINT('Ctrl Pts',(51.707657455628,15.042315526251,47.6812674158652));
#21868=CARTESIAN_POINT('Ctrl Pts',(51.6668956843904,15.2385243562794,47.6187972727124));
#21869=CARTESIAN_POINT('Ctrl Pts',(51.6071148687816,15.5262823101803,47.5271791708618));
#21870=CARTESIAN_POINT('Ctrl Pts',(51.5595992934775,15.8154197044411,47.4324063334734));
#21871=CARTESIAN_POINT('Ctrl Pts',(51.5244938097377,16.1049522263608,47.3345616995291));
#21872=CARTESIAN_POINT('Ctrl Pts',(51.4914040437863,16.3778601132494,47.2423351955216));
#21873=CARTESIAN_POINT('Ctrl Pts',(51.4693408708349,16.6511190964164,47.14737936348));
#21874=CARTESIAN_POINT('Ctrl Pts',(51.4584591192422,16.9238788974805,47.0497630002213));
#21875=CARTESIAN_POINT('Ctrl Pts',(51.4521604547632,17.0817599569435,46.9932598982535));
#21876=CARTESIAN_POINT('Ctrl Pts',(51.4496040028725,17.2394928872624,46.9358582204704));
#21877=CARTESIAN_POINT('Ctrl Pts',(51.4507739583774,17.3968661691267,46.8775869639482));
#21878=CARTESIAN_POINT('Ctrl Pts',(51.4528052320093,17.6700972420113,46.7764165635518));
#21879=CARTESIAN_POINT('Ctrl Pts',(51.4660705043716,17.942241477422,46.6726253927475));
#21880=CARTESIAN_POINT('Ctrl Pts',(51.4900980818398,18.2126518952105,46.5666544818487));
#21881=CARTESIAN_POINT('Ctrl Pts',(51.499926823275,18.3232662125019,46.5233059302001));
#21882=CARTESIAN_POINT('Ctrl Pts',(51.5115561621439,18.4335909686908,46.4795925387909));
#21883=CARTESIAN_POINT('Ctrl Pts',(51.5249529285916,18.5435841236212,46.4355440051706));
#21884=CARTESIAN_POINT('Ctrl Pts',(51.5638198253953,18.8626978902522,46.3077497484552));
#21885=CARTESIAN_POINT('Ctrl Pts',(51.6176238310752,19.1789902861077,46.17714612138));
#21886=CARTESIAN_POINT('Ctrl Pts',(51.6859043886847,19.4914647591776,46.0444546103236));
#21887=CARTESIAN_POINT('Ctrl Pts',(51.6935220631743,19.52632576362,46.0296509711305));
#21888=CARTESIAN_POINT('Ctrl Pts',(51.7013198745586,19.5611392285382,46.0148213612344));
#21889=CARTESIAN_POINT('Ctrl Pts',(51.7092971474407,19.5959037569241,45.9999667943664));
#21890=CARTESIAN_POINT('',(53.3864876685947,23.3160685634302,-44.2307692307677));
#21891=CARTESIAN_POINT('',(51.7092971560459,19.59597217608,-46.0001268989906));
#21892=CARTESIAN_POINT('Ctrl Pts',(53.3864876685928,23.3160685634274,-44.2307692307691));
#21893=CARTESIAN_POINT('Ctrl Pts',(52.930215177034,22.6766294615115,-44.5679874350866));
#21894=CARTESIAN_POINT('Ctrl Pts',(52.3546179283007,21.6420362564594,-45.0860447448006));
#21895=CARTESIAN_POINT('Ctrl Pts',(51.9005239862315,20.3541704296053,-45.6727447106325));
#21896=CARTESIAN_POINT('Ctrl Pts',(51.7529482282219,19.7864858334401,-45.9188374584652));
#21897=CARTESIAN_POINT('Ctrl Pts',(51.7092971610549,19.5959179422654,-46.));
#21898=CARTESIAN_POINT('',(71.6135123331932,23.3160685609228,-44.2307692320894));
#21899=CARTESIAN_POINT('Ctrl Pts',(71.6135123331932,23.3160685609229,-44.2307692320894));
#21900=CARTESIAN_POINT('Ctrl Pts',(71.1035100323559,24.0312794561666,-43.8537487425401));
#21901=CARTESIAN_POINT('Ctrl Pts',(69.681000122088,25.243380770632,-43.1696388054261));
#21902=CARTESIAN_POINT('Ctrl Pts',(66.9248798545188,26.2358932678842,-42.5648089417427));
#21903=CARTESIAN_POINT('Ctrl Pts',(63.9785719433368,26.5476372801886,-42.3700397756168));
#21904=CARTESIAN_POINT('Ctrl Pts',(61.0328912216257,26.5456758334602,-42.3710278989254));
#21905=CARTESIAN_POINT('Ctrl Pts',(58.0708968314258,26.2337622543912,-42.5667104493236));
#21906=CARTESIAN_POINT('Ctrl Pts',(55.3220849100951,25.2411372376895,-43.1704876695772));
#21907=CARTESIAN_POINT('Ctrl Pts',(53.9014731106537,24.038267655457,-43.8500649418989));
#21908=CARTESIAN_POINT('Ctrl Pts',(53.3864876685727,23.3160685633993,-44.2307692307839));
#21909=CARTESIAN_POINT('',(73.2907034369536,19.5966777272658,-46.0017752735852));
#21910=CARTESIAN_POINT('Ctrl Pts',(73.2907028389451,19.5959179422654,-46.));
#21911=CARTESIAN_POINT('Ctrl Pts',(73.2470092805887,19.7866035098537,-45.918783509084));
#21912=CARTESIAN_POINT('Ctrl Pts',(73.099528966838,20.3540492246571,-45.6728025929409));
#21913=CARTESIAN_POINT('Ctrl Pts',(72.6451832973973,21.6425621324406,-45.085801261871));
#21914=CARTESIAN_POINT('Ctrl Pts',(72.0694661900611,22.6771055141269,-44.5677393482618));
#21915=CARTESIAN_POINT('Ctrl Pts',(71.6135123331932,23.3160685609229,-44.2307692320894));
#21916=CARTESIAN_POINT('Ctrl Pts',(51.7092971560459,19.59597217608,-46.0001268989906));
#21917=CARTESIAN_POINT('Ctrl Pts',(51.6385518403573,19.2876757489281,-46.1318817425142));
#21918=CARTESIAN_POINT('Ctrl Pts',(51.5819245584145,18.9755341558142,-46.2616720942883));
#21919=CARTESIAN_POINT('Ctrl Pts',(51.5398657706017,18.6605076764483,-46.3887993378678));
#21920=CARTESIAN_POINT('Ctrl Pts',(51.5006578079912,18.3668342952929,-46.5073096533628));
#21921=CARTESIAN_POINT('Ctrl Pts',(51.4740774632621,18.0706621527521,-46.6235017985892));
#21922=CARTESIAN_POINT('Ctrl Pts',(51.4605290511144,17.7728302731532,-46.7367947468215));
#21923=CARTESIAN_POINT('Ctrl Pts',(51.4548236966847,17.6474106730525,-46.7845033946689));
#21924=CARTESIAN_POINT('Ctrl Pts',(51.4514287239645,17.5216967680026,-46.831698062969));
#21925=CARTESIAN_POINT('Ctrl Pts',(51.4503716252683,17.395751159985,-46.878336081621));
#21926=CARTESIAN_POINT('Ctrl Pts',(51.4493491529656,17.2739310344796,-46.9234464223063));
#21927=CARTESIAN_POINT('Ctrl Pts',(51.450513887619,17.1518941504805,-46.9680359923664));
#21928=CARTESIAN_POINT('Ctrl Pts',(51.4538566793357,17.0297349131611,-47.0120927720276));
#21929=CARTESIAN_POINT('Ctrl Pts',(51.4614578177917,16.7519583254358,-47.1122730137268));
#21930=CARTESIAN_POINT('Ctrl Pts',(51.4809069176557,16.4735134961054,-47.2097118040983));
#21931=CARTESIAN_POINT('Ctrl Pts',(51.5119283016989,16.1953334611301,-47.3043262340131));
#21932=CARTESIAN_POINT('Ctrl Pts',(51.540698040569,15.9373447474744,-47.3920732035939));
#21933=CARTESIAN_POINT('Ctrl Pts',(51.5794206384715,15.6795832662395,-47.4773912990985));
#21934=CARTESIAN_POINT('Ctrl Pts',(51.6278972920848,15.4227471168001,-47.560223409641));
#21935=CARTESIAN_POINT('Ctrl Pts',(51.6316912863093,15.4026460001803,-47.5667062116824));
#21936=CARTESIAN_POINT('Ctrl Pts',(51.6355450406446,15.3825505288608,-47.5731737896757));
#21937=CARTESIAN_POINT('Ctrl Pts',(51.6394584670014,15.3624610260131,-47.5796261178597));
#21938=CARTESIAN_POINT('Ctrl Pts',(51.6930034559185,15.0875888017152,-47.6679093279152));
#21939=CARTESIAN_POINT('Ctrl Pts',(51.7577243091049,14.8137957347893,-47.7533501196269));
#21940=CARTESIAN_POINT('Ctrl Pts',(51.8337259645455,14.5420228082065,-47.8358424485127));
#21941=CARTESIAN_POINT('Ctrl Pts',(51.9089081757662,14.2731801171894,-47.9174453512183));
#21942=CARTESIAN_POINT('Ctrl Pts',(51.9951298650042,14.0063139027635,-47.996162867403));
#21943=CARTESIAN_POINT('Ctrl Pts',(52.0925098200243,13.7423805361162,-48.0718777857805));
#21944=CARTESIAN_POINT('Ctrl Pts',(52.1693510364042,13.5341142565495,-48.1316234123319));
#21945=CARTESIAN_POINT('Ctrl Pts',(52.2531404764403,13.3276749982247,-48.1894991234461));
#21946=CARTESIAN_POINT('Ctrl Pts',(52.3439403254426,13.123554663829,-48.2454419686112));
#21947=CARTESIAN_POINT('Ctrl Pts',(52.4684627414818,12.8436251542427,-48.3221616803357));
#21948=CARTESIAN_POINT('Ctrl Pts',(52.6056097228968,12.5678248642511,-48.3953077688502));
#21949=CARTESIAN_POINT('Ctrl Pts',(52.7553388941879,12.2975172107946,-48.4646841952477));
#21950=CARTESIAN_POINT('Ctrl Pts',(52.9022559211048,12.0322863512615,-48.5327576255389));
#21951=CARTESIAN_POINT('Ctrl Pts',(53.0612868734049,11.7723444464564,-48.597201600181));
#21952=CARTESIAN_POINT('Ctrl Pts',(53.2323438982412,11.5189716531332,-48.6578426352013));
#21953=CARTESIAN_POINT('Ctrl Pts',(53.3005491093911,11.4179448471029,-48.6820219087615));
#21954=CARTESIAN_POINT('Ctrl Pts',(53.3706657391247,11.3179622781613,-48.7055967135365));
#21955=CARTESIAN_POINT('Ctrl Pts',(53.442686077265,11.2191043549872,-48.7285566222298));
#21956=CARTESIAN_POINT('Ctrl Pts',(53.6327962249655,10.9581517565786,-48.7891632750948));
#21957=CARTESIAN_POINT('Ctrl Pts',(53.8361749008966,10.7050379372868,-48.8454843564192));
#21958=CARTESIAN_POINT('Ctrl Pts',(54.0515222172661,10.4608362127091,-48.8977992033643));
#21959=CARTESIAN_POINT('Ctrl Pts',(54.2668695336356,10.2166344881313,-48.9501140503093));
#21960=CARTESIAN_POINT('Ctrl Pts',(54.4941848042496,9.98134567167982,-48.9984228060815));
#21961=CARTESIAN_POINT('Ctrl Pts',(54.7321208981018,9.75600333679323,-49.0430185827488));
#21962=CARTESIAN_POINT('Ctrl Pts',(54.9899860177656,9.51178680280687,-49.0913496076919));
#21963=CARTESIAN_POINT('Ctrl Pts',(55.2607617392154,9.27933854335903,-49.1353032978477));
#21964=CARTESIAN_POINT('Ctrl Pts',(55.5429655559212,9.05975496159557,-49.175295155659));
#21965=CARTESIAN_POINT('Ctrl Pts',(55.8271714636345,8.83861354720046,-49.215570735143));
#21966=CARTESIAN_POINT('Ctrl Pts',(56.1229687184755,8.63051923627181,-49.2518279919302));
#21967=CARTESIAN_POINT('Ctrl Pts',(56.4288895222584,8.43661493297673,-49.2844787968497));
#21968=CARTESIAN_POINT('Ctrl Pts',(56.7317789105064,8.24463205676346,-49.3168060600027));
#21969=CARTESIAN_POINT('Ctrl Pts',(57.0445928756025,8.06655867848375,-49.3455978623814));
#21970=CARTESIAN_POINT('Ctrl Pts',(57.3659431504788,7.90353716984582,-49.3712432917112));
#21971=CARTESIAN_POINT('Ctrl Pts',(57.6533784626551,7.75772077605303,-49.3941821299871));
#21972=CARTESIAN_POINT('Ctrl Pts',(57.9476441343405,7.6239468622901,-49.4146034724474));
#21973=CARTESIAN_POINT('Ctrl Pts',(58.2477651166754,7.50306255228726,-49.4327797488888));
#21974=CARTESIAN_POINT('Ctrl Pts',(58.4975711794082,7.40244435061056,-49.4479087945744));
#21975=CARTESIAN_POINT('Ctrl Pts',(58.7512496391542,7.31056607104857,-49.4615109231862));
#21976=CARTESIAN_POINT('Ctrl Pts',(59.008227698853,7.22798170126681,-49.4737304827943));
#21977=CARTESIAN_POINT('Ctrl Pts',(59.3398348334007,7.12141398006192,-49.4894987283474));
#21978=CARTESIAN_POINT('Ctrl Pts',(59.6769381471779,7.03032234664094,-49.5029647272155));
#21979=CARTESIAN_POINT('Ctrl Pts',(60.0179418759644,6.95485237030223,-49.5141055813766));
#21980=CARTESIAN_POINT('Ctrl Pts',(60.3605801711652,6.87902063636911,-49.52529983808));
#21981=CARTESIAN_POINT('Ctrl Pts',(60.7071563180931,6.81896148438955,-49.5341466700947));
#21982=CARTESIAN_POINT('Ctrl Pts',(61.0559988496054,6.7748238911007,-49.5406258175578));
#21983=CARTESIAN_POINT('Ctrl Pts',(61.4054206812244,6.73061300138095,-49.5471157245197));
#21984=CARTESIAN_POINT('Ctrl Pts',(61.7571162374109,6.70237741219055,-49.5512301065058));
#21985=CARTESIAN_POINT('Ctrl Pts',(62.1093548494777,6.69025593610002,-49.5529508633559));
#21986=CARTESIAN_POINT('Ctrl Pts',(62.2395261290315,6.68577639297575,-49.5535867763799));
#21987=CARTESIAN_POINT('Ctrl Pts',(62.3697710905136,6.68349739089685,-49.5538958114346));
#21988=CARTESIAN_POINT('Ctrl Pts',(62.5000007333252,6.6834252155456,-49.553877126063));
#21989=CARTESIAN_POINT('Ctrl Pts',(62.8097155764128,6.68325356662524,-49.5538326881239));
#21990=CARTESIAN_POINT('Ctrl Pts',(63.1194577152876,6.69569491589049,-49.5519170125618));
#21991=CARTESIAN_POINT('Ctrl Pts',(63.4280754364061,6.72060885415301,-49.5481478701364));
#21992=CARTESIAN_POINT('Ctrl Pts',(63.7370397386601,6.74555077104548,-49.5443744949221));
#21993=CARTESIAN_POINT('Ctrl Pts',(64.0448772410107,6.78299251361625,-49.5387434959438));
#21994=CARTESIAN_POINT('Ctrl Pts',(64.3504836874022,6.8328013328013,-49.531270901804));
#21995=CARTESIAN_POINT('Ctrl Pts',(64.4744054403698,6.85299853825798,-49.5282408054957));
#21996=CARTESIAN_POINT('Ctrl Pts',(64.5979609246064,6.87522937050882,-49.5249078823961));
#21997=CARTESIAN_POINT('Ctrl Pts',(64.7210788121852,6.89948581992488,-49.5212731237058));
#21998=CARTESIAN_POINT('Ctrl Pts',(65.0660710748529,6.96745553198623,-49.511088059216));
#21999=CARTESIAN_POINT('Ctrl Pts',(65.4076926497551,7.05106731795702,-49.4985686629476));
#22000=CARTESIAN_POINT('Ctrl Pts',(65.7441803838235,7.15037661535603,-49.4837109986881));
#22001=CARTESIAN_POINT('Ctrl Pts',(65.8269025362683,7.17479081536061,-49.4800583901576));
#22002=CARTESIAN_POINT('Ctrl Pts',(65.9093143931007,7.20015349248548,-49.4762645202421));
#22003=CARTESIAN_POINT('Ctrl Pts',(65.991389748064,7.2264649962254,-49.4723294411694));
#22004=CARTESIAN_POINT('Ctrl Pts',(66.3086238569636,7.32816308143608,-49.4571197438902));
#22005=CARTESIAN_POINT('Ctrl Pts',(66.6208301978817,7.44403920999634,-49.4397996750938));
#22006=CARTESIAN_POINT('Ctrl Pts',(66.926800548608,7.5731204565235,-49.420095339914));
#22007=CARTESIAN_POINT('Ctrl Pts',(67.2504549652406,7.70966216863315,-49.3992521598719));
#22008=CARTESIAN_POINT('Ctrl Pts',(67.5668631764223,7.86143247699165,-49.3756727657487));
#22009=CARTESIAN_POINT('Ctrl Pts',(67.874803872692,8.02722773016472,-49.3490305978458));
#22010=CARTESIAN_POINT('Ctrl Pts',(68.1861814260509,8.19487338699715,-49.3220910826785));
#22011=CARTESIAN_POINT('Ctrl Pts',(68.4889021298989,8.37685882175698,-49.2920202104801));
#22012=CARTESIAN_POINT('Ctrl Pts',(68.7817131552383,8.5719921786175,-49.258474106054));
#22013=CARTESIAN_POINT('Ctrl Pts',(69.0759255823596,8.7680594491983,-49.2247674490311));
#22014=CARTESIAN_POINT('Ctrl Pts',(69.3601341337972,8.97740094285658,-49.1875524295181));
#22015=CARTESIAN_POINT('Ctrl Pts',(69.6330655668965,9.19885896783842,-49.1464710786446));
#22016=CARTESIAN_POINT('Ctrl Pts',(69.7852554420347,9.32234664673131,-49.1235636194745));
#22017=CARTESIAN_POINT('Ctrl Pts',(69.9339387945752,9.44960263907514,-49.0994538173633));
#22018=CARTESIAN_POINT('Ctrl Pts',(70.0788929097391,9.58043280330667,-49.074077970154));
#22019=CARTESIAN_POINT('Ctrl Pts',(70.313741452996,9.79239831700799,-49.0329650928528));
#22020=CARTESIAN_POINT('Ctrl Pts',(70.5388860635807,10.0139710221455,-48.9884846155056));
#22021=CARTESIAN_POINT('Ctrl Pts',(70.753167983785,10.2441724186941,-48.940386756241));
#22022=CARTESIAN_POINT('Ctrl Pts',(70.9671407044207,10.4740416445564,-48.8923583001127));
#22023=CARTESIAN_POINT('Ctrl Pts',(71.1702817452254,10.7125139494238,-48.8407228352381));
#22024=CARTESIAN_POINT('Ctrl Pts',(71.3614834897188,10.9585938930529,-48.7852416133112));
#22025=CARTESIAN_POINT('Ctrl Pts',(71.4277417106301,11.0438693664019,-48.7660153919783));
#22026=CARTESIAN_POINT('Ctrl Pts',(71.4925666055447,11.130058281564,-48.7463274369041));
#22027=CARTESIAN_POINT('Ctrl Pts',(71.5559134725786,11.2171188605618,-48.7261681080344));
#22028=CARTESIAN_POINT('Ctrl Pts',(71.7401164260449,11.4702776438259,-48.6675478779967));
#22029=CARTESIAN_POINT('Ctrl Pts',(71.9118180082778,11.7308069507897,-48.6049411772279));
#22030=CARTESIAN_POINT('Ctrl Pts',(72.0709262012242,11.9973397782098,-48.5385160452646));
#22031=CARTESIAN_POINT('Ctrl Pts',(72.2333720073538,12.2694636657889,-48.4706975130492));
#22032=CARTESIAN_POINT('Ctrl Pts',(72.382690706961,12.5478447668155,-48.3988988215467));
#22033=CARTESIAN_POINT('Ctrl Pts',(72.5188369630493,12.8310332930558,-48.3233079989623));
#22034=CARTESIAN_POINT('Ctrl Pts',(72.5349764975393,12.8646040361503,-48.3143470423905));
#22035=CARTESIAN_POINT('Ctrl Pts',(72.5509309767563,12.8982423522582,-48.3053328036926));
#22036=CARTESIAN_POINT('Ctrl Pts',(72.5667003710721,12.9319458389031,-48.2962656029511));
#22037=CARTESIAN_POINT('Ctrl Pts',(72.7016360439085,13.2203400889478,-48.2186793109041));
#22038=CARTESIAN_POINT('Ctrl Pts',(72.8227250989957,13.5135818270332,-48.1371954523817));
#22039=CARTESIAN_POINT('Ctrl Pts',(72.9300166259904,13.8103594828784,-48.0519571049851));
#22040=CARTESIAN_POINT('Ctrl Pts',(73.0392119181037,14.1124031179207,-47.9652063008542));
#22041=CARTESIAN_POINT('Ctrl Pts',(73.1341161579519,14.4181097938983,-47.8745666597572));
#22042=CARTESIAN_POINT('Ctrl Pts',(73.2147473606732,14.726136307171,-47.7801737084575));
#22043=CARTESIAN_POINT('Ctrl Pts',(73.2592937260174,14.8963118860146,-47.7280243822338));
#22044=CARTESIAN_POINT('Ctrl Pts',(73.2994829882609,15.0671961837113,-47.6747291808002));
#22045=CARTESIAN_POINT('Ctrl Pts',(73.3353131082983,15.238566723947,-47.6203089053636));
#22046=CARTESIAN_POINT('Ctrl Pts',(73.4041812486989,15.5679535753776,-47.5157091115167));
#22047=CARTESIAN_POINT('Ctrl Pts',(73.4565608204754,15.8992610194355,-47.4069137146754));
#22048=CARTESIAN_POINT('Ctrl Pts',(73.4923097438172,16.2308818128794,-47.2940631567242));
#22049=CARTESIAN_POINT('Ctrl Pts',(73.5172428346201,16.4621707743967,-47.2153555217652));
#22050=CARTESIAN_POINT('Ctrl Pts',(73.534085099451,16.693612313661,-47.134675100752));
#22051=CARTESIAN_POINT('Ctrl Pts',(73.5427735626241,16.9246603998039,-47.0520669694327));
#22052=CARTESIAN_POINT('Ctrl Pts',(73.5487224225862,17.0828555468144,-46.9955064252772));
#22053=CARTESIAN_POINT('Ctrl Pts',(73.55102694222,17.2408810307338,-46.9380367751146));
#22054=CARTESIAN_POINT('Ctrl Pts',(73.5496650158222,17.3985337770098,-46.8796814170754));
#22055=CARTESIAN_POINT('Ctrl Pts',(73.5470374585348,17.7026923739799,-46.7670967381138));
#22056=CARTESIAN_POINT('Ctrl Pts',(73.5307595350488,18.005463438459,-46.6512144067101));
#22057=CARTESIAN_POINT('Ctrl Pts',(73.5012734326613,18.3059881853662,-46.5326475787612));
#22058=CARTESIAN_POINT('Ctrl Pts',(73.4934571778605,18.3856520882075,-46.501217567226));
#22059=CARTESIAN_POINT('Ctrl Pts',(73.4847130769512,18.4651581483415,-46.4695989899252));
#22060=CARTESIAN_POINT('Ctrl Pts',(73.4750499542682,18.5444903963155,-46.4378034063969));
#22061=CARTESIAN_POINT('Ctrl Pts',(73.4381093912684,18.8477648139483,-46.3162540072046));
#22062=CARTESIAN_POINT('Ctrl Pts',(73.3876764007721,19.1484717215781,-46.1921283391257));
#22063=CARTESIAN_POINT('Ctrl Pts',(73.3241452988119,19.4457621095765,-46.0660620702451));
#22064=CARTESIAN_POINT('Ctrl Pts',(73.3133737523194,19.4961669843122,-46.0446878356655));
#22065=CARTESIAN_POINT('Ctrl Pts',(73.3022257825704,19.5464735904137,-46.0232578551976));
#22066=CARTESIAN_POINT('Ctrl Pts',(73.2907034369536,19.5966777272658,-46.0017752735852));
#22067=CARTESIAN_POINT('Ctrl Pts',(55.0359921611649,23.1177228316711,46.));
#22068=CARTESIAN_POINT('Ctrl Pts',(54.6885805899455,22.6146358479788,46.));
#22069=CARTESIAN_POINT('Ctrl Pts',(54.1137702212827,21.7689600531191,46.));
#22070=CARTESIAN_POINT('Ctrl Pts',(53.267851387655,20.6527649215947,46.0000000000001));
#22071=CARTESIAN_POINT('Ctrl Pts',(52.6132688313215,19.9575001862921,45.9999999999999));
#22072=CARTESIAN_POINT('Ctrl Pts',(52.0600422917726,19.6355082498452,46.0000000000001));
#22073=CARTESIAN_POINT('Ctrl Pts',(51.7092971610549,19.5959179422654,46.));
#22074=CARTESIAN_POINT('Ctrl Pts',(54.8498454495129,22.8208715049056,45.1947514602968));
#22075=CARTESIAN_POINT('Ctrl Pts',(54.4276728878709,22.4046326878925,45.2688266414859));
#22076=CARTESIAN_POINT('Ctrl Pts',(53.7584764072867,21.670812023264,45.4340456995033));
#22077=CARTESIAN_POINT('Ctrl Pts',(52.9162294593297,20.6402827270753,45.7053535607057));
#22078=CARTESIAN_POINT('Ctrl Pts',(52.3583769742476,19.9751884160731,45.8895956767591));
#22079=CARTESIAN_POINT('Ctrl Pts',(51.9502746726906,19.6521457104047,45.9816693098607));
#22080=CARTESIAN_POINT('Ctrl Pts',(51.7092971610549,19.5959179422654,46.));
#22081=CARTESIAN_POINT('Ctrl Pts',(54.1372439325421,22.9065587328174,44.4304270626387));
#22082=CARTESIAN_POINT('Ctrl Pts',(53.7472447505792,22.4964832086346,44.6462611267445));
#22083=CARTESIAN_POINT('Ctrl Pts',(53.1541646175812,21.7560680203378,45.0210196472744));
#22084=CARTESIAN_POINT('Ctrl Pts',(52.4850075211232,20.6995709152847,45.5168050506341));
#22085=CARTESIAN_POINT('Ctrl Pts',(52.0911343848321,20.0136370147741,45.8210758339952));
#22086=CARTESIAN_POINT('Ctrl Pts',(51.840758511164,19.6707821067247,45.968114937896));
#22087=CARTESIAN_POINT('Ctrl Pts',(51.7092971610549,19.5959179422654,46.));
#22088=CARTESIAN_POINT('Ctrl Pts',(53.3864876668068,23.3160685609229,44.2307692320894));
#22089=CARTESIAN_POINT('Ctrl Pts',(53.0439951189989,22.8358340303902,44.4839588612342));
#22090=CARTESIAN_POINT('Ctrl Pts',(52.5423502486883,21.9908524941898,44.9125177602508));
#22091=CARTESIAN_POINT('Ctrl Pts',(52.0530341102106,20.8197959816443,45.4633470605684));
#22092=CARTESIAN_POINT('Ctrl Pts',(51.8239020992648,20.0709136872745,45.7962695577249));
#22093=CARTESIAN_POINT('Ctrl Pts',(51.7312389779497,19.6914330268016,45.959302575355));
#22094=CARTESIAN_POINT('Ctrl Pts',(51.7092971610549,19.5959179422654,46.));
#22095=CARTESIAN_POINT('Origin',(53.3864876668068,24.2487113033598,46.000000001373));
#22096=CARTESIAN_POINT('Ctrl Pts',(55.035992162965,23.1177228342965,46.));
#22097=CARTESIAN_POINT('Ctrl Pts',(54.3299192064178,22.0879417672428,46.));
#22098=CARTESIAN_POINT('Ctrl Pts',(53.8230715593574,21.3650115665077,46.));
#22099=CARTESIAN_POINT('Ctrl Pts',(53.0821556643503,20.4538645006679,46.));
#22100=CARTESIAN_POINT('Ctrl Pts',(52.7982587176799,20.151721721479,46.));
#22101=CARTESIAN_POINT('Ctrl Pts',(52.3967587125637,19.8400027811804,46.));
#22102=CARTESIAN_POINT('Ctrl Pts',(52.2554329542124,19.7480371194989,46.0000000000325));
#22103=CARTESIAN_POINT('Ctrl Pts',(52.0414383936788,19.6565556786848,46.0000000000325));
#22104=CARTESIAN_POINT('Ctrl Pts',(51.9738964717323,19.6337322451885,46.));
#22105=CARTESIAN_POINT('Ctrl Pts',(51.8404098310991,19.6038714213037,46.));
#22106=CARTESIAN_POINT('Ctrl Pts',(51.7751374400014,19.5959179422654,46.));
#22107=CARTESIAN_POINT('Ctrl Pts',(51.7092971610549,19.5959179422654,46.));
#22108=CARTESIAN_POINT('Ctrl Pts',(69.9640078370513,23.1177228342728,46.));
#22109=CARTESIAN_POINT('Ctrl Pts',(69.542232429734,23.7328665315065,46.));
#22110=CARTESIAN_POINT('Ctrl Pts',(68.5372497203374,24.8762781693712,46.));
#22111=CARTESIAN_POINT('Ctrl Pts',(66.5003162911619,26.2518765973163,46.));
#22112=CARTESIAN_POINT('Ctrl Pts',(63.9229202346607,27.0854099302792,46.));
#22113=CARTESIAN_POINT('Ctrl Pts',(61.0682561393548,27.0809097910938,46.));
#22114=CARTESIAN_POINT('Ctrl Pts',(58.4978723140799,26.2506120287296,46.));
#22115=CARTESIAN_POINT('Ctrl Pts',(56.4626291503929,24.8770023535894,46.));
#22116=CARTESIAN_POINT('Ctrl Pts',(55.4536863537726,23.7269142298698,46.));
#22117=CARTESIAN_POINT('Ctrl Pts',(55.0359921615024,23.1177228321634,46.));
#22118=CARTESIAN_POINT('Ctrl Pts',(70.0200075221065,23.036049382692,45.7722265692886));
#22119=CARTESIAN_POINT('Ctrl Pts',(69.5701845212888,23.6267219749651,45.7450333341526));
#22120=CARTESIAN_POINT('Ctrl Pts',(68.5033702547963,24.6932485864254,45.7248984528665));
#22121=CARTESIAN_POINT('Ctrl Pts',(66.4423862476702,25.9202843643973,45.7851490895574));
#22122=CARTESIAN_POINT('Ctrl Pts',(63.9082001948719,26.6583896707281,45.8854558492519));
#22123=CARTESIAN_POINT('Ctrl Pts',(61.0833863606388,26.6544061954588,45.8839043324688));
#22124=CARTESIAN_POINT('Ctrl Pts',(58.5556906298045,25.9185765932678,45.7844483918357));
#22125=CARTESIAN_POINT('Ctrl Pts',(56.4966824739014,24.6938781056256,45.7240522007472));
#22126=CARTESIAN_POINT('Ctrl Pts',(55.4254628658836,23.6210064625855,45.7452964634328));
#22127=CARTESIAN_POINT('Ctrl Pts',(54.9799924763511,23.0360493806665,45.772226569382));
#22128=CARTESIAN_POINT('Ctrl Pts',(70.2092197650832,22.9256684193351,45.3167264994702));
#22129=CARTESIAN_POINT('Ctrl Pts',(69.7158291105167,23.4853279772436,45.2164752999052));
#22130=CARTESIAN_POINT('Ctrl Pts',(68.535014472362,24.4361203670811,45.0981257954975));
#22131=CARTESIAN_POINT('Ctrl Pts',(66.383710902278,25.3846466842565,45.1588861842134));
#22132=CARTESIAN_POINT('Ctrl Pts',(63.8865686721771,25.8842035797987,45.3602142350906));
#22133=CARTESIAN_POINT('Ctrl Pts',(61.1051010280161,25.8825087356241,45.3567819163901));
#22134=CARTESIAN_POINT('Ctrl Pts',(58.6143395050501,25.3831984355184,45.1570202136384));
#22135=CARTESIAN_POINT('Ctrl Pts',(56.4652796759868,24.4374218336232,45.0958734343921));
#22136=CARTESIAN_POINT('Ctrl Pts',(55.279396703872,23.479912555679,45.2174453583462));
#22137=CARTESIAN_POINT('Ctrl Pts',(54.7907802332251,22.9256684174159,45.316726499814));
#22138=CARTESIAN_POINT('Ctrl Pts',(70.6459692050112,22.9403123749432,44.776430516514));
#22139=CARTESIAN_POINT('Ctrl Pts',(70.1274758860988,23.5168125343884,44.5569401518289));
#22140=CARTESIAN_POINT('Ctrl Pts',(68.8339836677725,24.4521830465394,44.2171354911649));
#22141=CARTESIAN_POINT('Ctrl Pts',(66.4852650826246,25.2255541487752,44.0484187526542));
#22142=CARTESIAN_POINT('Ctrl Pts',(63.8933590415983,25.4907416731797,44.1400917531453));
#22143=CARTESIAN_POINT('Ctrl Pts',(61.0969988006743,25.4920128625193,44.1369164712371));
#22144=CARTESIAN_POINT('Ctrl Pts',(58.5131163976547,25.2255225866375,44.0466798604088));
#22145=CARTESIAN_POINT('Ctrl Pts',(56.1663207696582,24.4550752730798,44.2144948710689));
#22146=CARTESIAN_POINT('Ctrl Pts',(54.8675070278469,23.5112341585235,44.5590640016228));
#22147=CARTESIAN_POINT('Ctrl Pts',(54.3540307932109,22.9403123729663,44.7764305172667));
#22148=CARTESIAN_POINT('Ctrl Pts',(71.13576024646,23.0841835154325,44.412288853233));
#22149=CARTESIAN_POINT('Ctrl Pts',(70.6147355135831,23.7210088220381,44.0947795647742));
#22150=CARTESIAN_POINT('Ctrl Pts',(69.2492273035993,24.7560226484019,43.5531210449959));
#22151=CARTESIAN_POINT('Ctrl Pts',(66.6913084652411,25.5729841387648,43.1242832122387));
#22152=CARTESIAN_POINT('Ctrl Pts',(63.9257521800277,25.7932760987112,43.0406381319293));
#22153=CARTESIAN_POINT('Ctrl Pts',(61.0627975487631,25.7956751380647,43.0388168513456));
#22154=CARTESIAN_POINT('Ctrl Pts',(58.3074986944687,25.5736178460725,43.1233746593592));
#22155=CARTESIAN_POINT('Ctrl Pts',(55.7509094065862,24.7598092206675,43.5507965518109));
#22156=CARTESIAN_POINT('Ctrl Pts',(54.3802229056199,23.7148467232691,44.0978518729798));
#22157=CARTESIAN_POINT('Ctrl Pts',(53.8642397517534,23.0841835132488,44.4122888543217));
#22158=CARTESIAN_POINT('Ctrl Pts',(71.4542425639415,23.2306116904396,44.2758174708167));
#22159=CARTESIAN_POINT('Ctrl Pts',(70.9372237337292,23.9223005711455,43.9129480259072));
#22160=CARTESIAN_POINT('Ctrl Pts',(69.5371396621711,25.0636258970674,43.2733988845769));
#22161=CARTESIAN_POINT('Ctrl Pts',(66.8466481816036,25.991977143232,42.7149637246248));
#22162=CARTESIAN_POINT('Ctrl Pts',(63.9528070871081,26.2647811407212,42.546738631874));
#22163=CARTESIAN_POINT('Ctrl Pts',(61.0345041648995,26.2670739944513,42.5455363906498));
#22164=CARTESIAN_POINT('Ctrl Pts',(58.1524504628798,25.9925148535544,42.714387867757));
#22165=CARTESIAN_POINT('Ctrl Pts',(55.4628430152718,25.0675639103996,43.2712020277055));
#22166=CARTESIAN_POINT('Ctrl Pts',(54.0577734476554,23.9156075971566,43.9164592516275));
#22167=CARTESIAN_POINT('Ctrl Pts',(53.5457574342856,23.2306116880677,44.275817472061));
#22168=CARTESIAN_POINT('Ctrl Pts',(71.6135123314272,23.3160685633993,44.2307692307839));
#22169=CARTESIAN_POINT('Ctrl Pts',(71.0985268893462,24.038267655457,43.8500649418989));
#22170=CARTESIAN_POINT('Ctrl Pts',(69.681226557465,25.239555364586,43.1717497595138));
#22171=CARTESIAN_POINT('Ctrl Pts',(66.9244886027247,26.2356604580669,42.5652091566662));
#22172=CARTESIAN_POINT('Ctrl Pts',(63.9663874943631,26.5460492373018,42.3707472230138));
#22173=CARTESIAN_POINT('Ctrl Pts',(61.020309894555,26.5481066493621,42.3696710366589));
#22174=CARTESIAN_POINT('Ctrl Pts',(58.0747486677894,26.2360703120526,42.564673612103));
#22175=CARTESIAN_POINT('Ctrl Pts',(55.3186828044349,25.2435158958716,43.1695330127632));
#22176=CARTESIAN_POINT('Ctrl Pts',(53.8964899676441,24.0312794561666,43.8537487425402));
#22177=CARTESIAN_POINT('Ctrl Pts',(53.3864876668068,23.3160685609229,44.2307692320894));
#22178=CARTESIAN_POINT('Origin',(71.6135123314049,24.2487113059679,45.9999999999981));
#22179=CARTESIAN_POINT('Ctrl Pts',(73.2907035679191,19.5959179422654,46.));
#22180=CARTESIAN_POINT('Ctrl Pts',(73.2853132736892,19.5959179422654,46.));
#22181=CARTESIAN_POINT('Ctrl Pts',(73.2800921964744,19.5959613316258,46.));
#22182=CARTESIAN_POINT('Ctrl Pts',(73.190737153897,19.5979267180889,46.));
#22183=CARTESIAN_POINT('Ctrl Pts',(73.0919541682948,19.6164825507722,46.));
#22184=CARTESIAN_POINT('Ctrl Pts',(72.9349512659537,19.6613683597688,46.));
#22185=CARTESIAN_POINT('Ctrl Pts',(72.7366254879835,19.7544322191794,46.));
#22186=CARTESIAN_POINT('Ctrl Pts',(72.5187524776661,19.8974562011792,46.));
#22187=CARTESIAN_POINT('Ctrl Pts',(72.3059356178939,20.0751969944156,46.));
#22188=CARTESIAN_POINT('Ctrl Pts',(72.1177575559123,20.2549369737277,46.));
#22189=CARTESIAN_POINT('Ctrl Pts',(71.9467703806141,20.4356656328949,46.));
#22190=CARTESIAN_POINT('Ctrl Pts',(71.7871832912953,20.6165764559116,46.));
#22191=CARTESIAN_POINT('Ctrl Pts',(71.6363028797942,20.7973306481917,46.));
#22192=CARTESIAN_POINT('Ctrl Pts',(71.4916909653841,20.977997589463,46.));
#22193=CARTESIAN_POINT('Ctrl Pts',(71.3520460598813,21.1584331287946,46.));
#22194=CARTESIAN_POINT('Ctrl Pts',(71.2162849549212,21.3385618577325,46.));
#22195=CARTESIAN_POINT('Ctrl Pts',(71.1057852053627,21.488374549024,46.));
#22196=CARTESIAN_POINT('Ctrl Pts',(71.0186156532208,21.6080221976867,46.));
#22197=CARTESIAN_POINT('Ctrl Pts',(70.8890085638933,21.7872920165661,46.));
#22198=CARTESIAN_POINT('Ctrl Pts',(70.7410429419584,21.9958939832604,46.));
#22199=CARTESIAN_POINT('Ctrl Pts',(70.5744311075321,22.2333786866411,46.));
#22200=CARTESIAN_POINT('Ctrl Pts',(70.409440490942,22.4703098380079,46.));
#22201=CARTESIAN_POINT('Ctrl Pts',(70.2056431651792,22.765428405125,46.));
#22202=CARTESIAN_POINT('Ctrl Pts',(70.0444070209061,23.0004636239141,46.));
#22203=CARTESIAN_POINT('Ctrl Pts',(69.9640078370348,23.1177228342968,46.));
#22204=CARTESIAN_POINT('Ctrl Pts',(73.2907035679191,19.5959179422654,46.));
#22205=CARTESIAN_POINT('Ctrl Pts',(73.2862490793568,19.5960900665757,45.9999175533143));
#22206=CARTESIAN_POINT('Ctrl Pts',(73.2820811790803,19.5963336271153,45.9998440681509));
#22207=CARTESIAN_POINT('Ctrl Pts',(73.208253200484,19.6010450092914,45.9982213945468));
#22208=CARTESIAN_POINT('Ctrl Pts',(73.1274794573141,19.6220399195827,45.9943050481736));
#22209=CARTESIAN_POINT('Ctrl Pts',(72.9963653350095,19.6695017870272,45.9858046677887));
#22210=CARTESIAN_POINT('Ctrl Pts',(72.8294716734784,19.764069356512,45.9701218125784));
#22211=CARTESIAN_POINT('Ctrl Pts',(72.6414650292326,19.9063529120636,45.9471817238329));
#22212=CARTESIAN_POINT('Ctrl Pts',(72.4536342973198,20.081311370936,45.9196661796449));
#22213=CARTESIAN_POINT('Ctrl Pts',(72.2835895740479,20.2570788809575,45.8924066669206));
#22214=CARTESIAN_POINT('Ctrl Pts',(72.1258636290523,20.4329402115168,45.8655395060906));
#22215=CARTESIAN_POINT('Ctrl Pts',(71.9757248574748,20.6082090575464,45.8391421338054));
#22216=CARTESIAN_POINT('Ctrl Pts',(71.8311830958701,20.7826098635032,45.8132826543535));
#22217=CARTESIAN_POINT('Ctrl Pts',(71.6902708461682,20.9562249829189,45.7879723330246));
#22218=CARTESIAN_POINT('Ctrl Pts',(71.5520244073844,21.1289170402946,45.7632628720577));
#22219=CARTESIAN_POINT('Ctrl Pts',(71.4156157450574,21.3006067154702,45.7392000949141));
#22220=CARTESIAN_POINT('Ctrl Pts',(71.3030395865729,21.4428000487426,45.7197248605149));
#22221=CARTESIAN_POINT('Ctrl Pts',(71.2133703207735,21.5559942629584,45.7045133261289));
#22222=CARTESIAN_POINT('Ctrl Pts',(71.0792059015168,21.7252227168858,45.6820761723759));
#22223=CARTESIAN_POINT('Ctrl Pts',(70.9236830208857,21.9210467851455,45.6570406101074));
#22224=CARTESIAN_POINT('Ctrl Pts',(70.7457968935764,22.1424153277308,45.630177451962));
#22225=CARTESIAN_POINT('Ctrl Pts',(70.5678883520528,22.3622036711249,45.6045437380644));
#22226=CARTESIAN_POINT('Ctrl Pts',(70.3450747297217,22.6339353529314,45.5749261951409));
#22227=CARTESIAN_POINT('Ctrl Pts',(70.165943219464,22.8481046901869,45.5540871152153));
#22228=CARTESIAN_POINT('Ctrl Pts',(70.0760072071431,22.9543759311333,45.5444531385751));
#22229=CARTESIAN_POINT('Ctrl Pts',(73.2907035679191,19.5959179422654,46.));
#22230=CARTESIAN_POINT('Ctrl Pts',(73.2880504840915,19.5964289578032,45.9997781423769));
#22231=CARTESIAN_POINT('Ctrl Pts',(73.2853846053994,19.5969457764203,45.9995692096135));
#22232=CARTESIAN_POINT('Ctrl Pts',(73.2411647337054,19.6070786822663,45.995310811962));
#22233=CARTESIAN_POINT('Ctrl Pts',(73.1895361350525,19.6323355913422,45.9857343837773));
#22234=CARTESIAN_POINT('Ctrl Pts',(73.1063585625323,19.6861977169776,45.96540896875));
#22235=CARTESIAN_POINT('Ctrl Pts',(72.9951136441404,19.7861798679065,45.9282889331739));
#22236=CARTESIAN_POINT('Ctrl Pts',(72.8650301145033,19.9324850330593,45.8739794495604));
#22237=CARTESIAN_POINT('Ctrl Pts',(72.7278523001271,20.1091863830438,45.8082212986075));
#22238=CARTESIAN_POINT('Ctrl Pts',(72.599008386305,20.2853439277712,45.7422966248579));
#22239=CARTESIAN_POINT('Ctrl Pts',(72.4749524884831,20.4604229392962,45.6764333722182));
#22240=CARTESIAN_POINT('Ctrl Pts',(72.3531838593419,20.634045289074,45.6107610623116));
#22241=CARTESIAN_POINT('Ctrl Pts',(72.2325138280896,20.8059659224486,45.545403805715));
#22242=CARTESIAN_POINT('Ctrl Pts',(72.1118213239367,20.9763160140027,45.4803379945738));
#22243=CARTESIAN_POINT('Ctrl Pts',(71.9905611813765,21.1449425524697,45.4156563653195));
#22244=CARTESIAN_POINT('Ctrl Pts',(71.8682925794356,21.3117528991958,45.3514312058611));
#22245=CARTESIAN_POINT('Ctrl Pts',(71.7653253439371,21.4491702215447,45.2983550050255));
#22246=CARTESIAN_POINT('Ctrl Pts',(71.682174619526,21.5581056496617,45.2561979636126));
#22247=CARTESIAN_POINT('Ctrl Pts',(71.5566443241353,21.7204926694612,45.1932855292725));
#22248=CARTESIAN_POINT('Ctrl Pts',(71.4078049567651,21.9069447194497,45.1208830261352));
#22249=CARTESIAN_POINT('Ctrl Pts',(71.2337951661038,22.1155847374877,45.0398130889285));
#22250=CARTESIAN_POINT('Ctrl Pts',(71.0572027402818,22.3211899834939,44.9599661565235));
#22251=CARTESIAN_POINT('Ctrl Pts',(70.8314760697034,22.5723353005728,44.8626519726254));
#22252=CARTESIAN_POINT('Ctrl Pts',(70.6454769955238,22.7666605685381,44.787912840376));
#22253=CARTESIAN_POINT('Ctrl Pts',(70.5510931890894,22.8620875206656,44.7514416370933));
#22254=CARTESIAN_POINT('Ctrl Pts',(73.2907035679191,19.5959179422654,46.));
#22255=CARTESIAN_POINT('Ctrl Pts',(73.2897792520886,19.5967541971494,45.9996437628225));
#22256=CARTESIAN_POINT('Ctrl Pts',(73.288766733936,19.5975749243332,45.9992940960059));
#22257=CARTESIAN_POINT('Ctrl Pts',(73.2730749026927,19.6130270044881,45.9927106906892));
#22258=CARTESIAN_POINT('Ctrl Pts',(73.251756086113,19.6437149190236,45.9796188466631));
#22259=CARTESIAN_POINT('Ctrl Pts',(73.216079179159,19.7062122776897,45.9528815794702));
#22260=CARTESIAN_POINT('Ctrl Pts',(73.1625244070959,19.8168600337209,45.9053443493137));
#22261=CARTESIAN_POINT('Ctrl Pts',(73.0934344901874,19.975480126619,45.8366125412608));
#22262=CARTESIAN_POINT('Ctrl Pts',(73.0131490016378,20.1651666288159,45.7534836745954));
#22263=CARTESIAN_POINT('Ctrl Pts',(72.9327871582964,20.3538190600323,45.6698774417649));
#22264=CARTESIAN_POINT('Ctrl Pts',(72.8511054586688,20.5411597726202,45.5859293751855));
#22265=CARTESIAN_POINT('Ctrl Pts',(72.7674694094519,20.7270595237571,45.5017127400763));
#22266=CARTESIAN_POINT('Ctrl Pts',(72.6815224957815,20.9113376828887,45.417327487362));
#22267=CARTESIAN_POINT('Ctrl Pts',(72.5928892631333,21.0942091320849,45.3326926851353));
#22268=CARTESIAN_POINT('Ctrl Pts',(72.5014236904482,21.2755404995838,45.24788633318));
#22269=CARTESIAN_POINT('Ctrl Pts',(72.4070183371161,21.4552564835779,45.1629622322214));
#22270=CARTESIAN_POINT('Ctrl Pts',(72.3258429327874,21.603596996729,45.0921463541392));
#22271=CARTESIAN_POINT('Ctrl Pts',(72.2593780519087,21.7213758855668,45.0354955830711));
#22272=CARTESIAN_POINT('Ctrl Pts',(72.1581530560203,21.8971298392077,44.9505368909156));
#22273=CARTESIAN_POINT('Ctrl Pts',(72.0355742524663,22.0994507797852,44.8515128507767));
#22274=CARTESIAN_POINT('Ctrl Pts',(71.8893300919241,22.3266244145461,44.7387188968997));
#22275=CARTESIAN_POINT('Ctrl Pts',(71.7390041704018,22.5509982091827,44.6262592382376));
#22276=CARTESIAN_POINT('Ctrl Pts',(71.5434859051336,22.8260292236067,44.4864687330478));
#22277=CARTESIAN_POINT('Ctrl Pts',(71.3791052619253,23.0398714682527,44.3758130784414));
#22278=CARTESIAN_POINT('Ctrl Pts',(71.2949727964356,23.1451548175056,44.320865710836));
#22279=CARTESIAN_POINT('Ctrl Pts',(73.2907035679191,19.5959179422654,46.));
#22280=CARTESIAN_POINT('Ctrl Pts',(73.2904808728319,19.5968857094338,45.9995877329126));
#22281=CARTESIAN_POINT('Ctrl Pts',(73.2902587582729,19.5978534806893,45.9991754285667));
#22282=CARTESIAN_POINT('Ctrl Pts',(73.2862090342068,19.6154867193585,45.9916623858903));
#22283=CARTESIAN_POINT('Ctrl Pts',(73.278471643703,19.6487953456216,45.977449084781));
#22284=CARTESIAN_POINT('Ctrl Pts',(73.2626675329748,19.7153221034526,45.9489756536103));
#22285=CARTESIAN_POINT('Ctrl Pts',(73.2341485984696,19.8314987172849,45.8990281581236));
#22286=CARTESIAN_POINT('Ctrl Pts',(73.1909498335265,19.9967609507555,45.8273396719058));
#22287=CARTESIAN_POINT('Ctrl Pts',(73.1352131070871,20.1938738237251,45.7408225076835));
#22288=CARTESIAN_POINT('Ctrl Pts',(73.0755852718533,20.3897951762557,45.6538223879631));
#22289=CARTESIAN_POINT('Ctrl Pts',(73.0121109467716,20.5844107113345,45.5664035981079));
#22290=CARTESIAN_POINT('Ctrl Pts',(72.9448178995343,20.7776647362872,45.4786056970811));
#22291=CARTESIAN_POINT('Ctrl Pts',(72.8737703412485,20.969415619956,45.3905097941917));
#22292=CARTESIAN_POINT('Ctrl Pts',(72.7988814082159,21.1599111909158,45.302017540834));
#22293=CARTESIAN_POINT('Ctrl Pts',(72.7201916785671,21.3490306679124,45.2131989345674));
#22294=CARTESIAN_POINT('Ctrl Pts',(72.6377280503905,21.5367060266982,45.1241021330032));
#22295=CARTESIAN_POINT('Ctrl Pts',(72.5658930280084,21.6918256295662,45.0496717620424));
#22296=CARTESIAN_POINT('Ctrl Pts',(72.5065732598677,21.8151167092688,44.990045399374));
#22297=CARTESIAN_POINT('Ctrl Pts',(72.4157517404387,21.9992281010938,44.9005387053819));
#22298=CARTESIAN_POINT('Ctrl Pts',(72.3044475744177,22.211560601306,44.7959596617311));
#22299=CARTESIAN_POINT('Ctrl Pts',(72.1700773346563,22.4505358369901,44.6764670164254));
#22300=CARTESIAN_POINT('Ctrl Pts',(72.0309897669014,22.6869514584429,44.557072726346));
#22301=CARTESIAN_POINT('Ctrl Pts',(71.8483990288815,22.9774859633438,44.4081667977607));
#22302=CARTESIAN_POINT('Ctrl Pts',(71.6932714543115,23.2042169236777,44.2897313638428));
#22303=CARTESIAN_POINT('Ctrl Pts',(71.6135123314072,23.3160685634275,44.2307692307691));
#22304=CARTESIAN_POINT('Ctrl Pts',(73.2907028389451,19.5959179422654,46.));
#22305=CARTESIAN_POINT('Ctrl Pts',(73.1782488824317,19.5959179422654,46.));
#22306=CARTESIAN_POINT('Ctrl Pts',(73.0679692680469,19.6191095759631,46.0000000000001));
#22307=CARTESIAN_POINT('Ctrl Pts',(72.7990151985813,19.7161705537826,46.0000000000001));
#22308=CARTESIAN_POINT('Ctrl Pts',(72.6442834670101,19.8115682299362,45.999999999991));
#22309=CARTESIAN_POINT('Ctrl Pts',(72.2391188325035,20.1170685085798,45.999999999991));
#22310=CARTESIAN_POINT('Ctrl Pts',(71.9632856619516,20.4043146233181,46.));
#22311=CARTESIAN_POINT('Ctrl Pts',(71.2192192201258,21.3045670772791,46.));
#22312=CARTESIAN_POINT('Ctrl Pts',(70.6968197820516,22.0489439500589,46.));
#22313=CARTESIAN_POINT('Ctrl Pts',(69.964007837035,23.1177228342965,46.));
#22314=CARTESIAN_POINT('Ctrl Pts',(55.035992162965,23.1177228342965,46.));
#22315=CARTESIAN_POINT('Ctrl Pts',(54.0296627127653,21.6500288723272,46.9446698131654));
#22316=CARTESIAN_POINT('Ctrl Pts',(52.8893156673895,18.1414957976349,48.915242890626));
#22317=CARTESIAN_POINT('Ctrl Pts',(54.5395958207989,12.4855237992675,50.8957649600243));
#22318=CARTESIAN_POINT('Ctrl Pts',(59.4315484638286,8.79278472652513,51.5632592674646));
#22319=CARTESIAN_POINT('Ctrl Pts',(65.5663223673701,8.80057359018861,51.5646626464224));
#22320=CARTESIAN_POINT('Ctrl Pts',(70.463129301692,12.4814952571317,50.8974409168532));
#22321=CARTESIAN_POINT('Ctrl Pts',(72.1120278968484,18.1410701930242,48.9161444008817));
#22322=CARTESIAN_POINT('Ctrl Pts',(70.9703446072329,21.6500181963829,46.944676684654));
#22323=CARTESIAN_POINT('Ctrl Pts',(69.964007837035,23.1177228342965,46.));
#22324=CARTESIAN_POINT('Ctrl Pts',(54.9799924779109,23.0360493827148,45.7722265692876));
#22325=CARTESIAN_POINT('Ctrl Pts',(53.9836364614215,21.5483875117231,46.7011217010093));
#22326=CARTESIAN_POINT('Ctrl Pts',(52.8947746067151,18.0181392478017,48.6325382140834));
#22327=CARTESIAN_POINT('Ctrl Pts',(54.5878793708661,12.4419398028121,50.5700934772302));
#22328=CARTESIAN_POINT('Ctrl Pts',(59.4430893598328,8.79596203843427,51.238449475546));
#22329=CARTESIAN_POINT('Ctrl Pts',(65.55434777324,8.80321749148772,51.2397703452684));
#22330=CARTESIAN_POINT('Ctrl Pts',(70.41476928952,12.438794404978,50.5716603603405));
#22331=CARTESIAN_POINT('Ctrl Pts',(72.1066202548239,18.0180329314669,48.6333855335872));
#22332=CARTESIAN_POINT('Ctrl Pts',(71.0163707860304,21.5483766905331,46.7011284577535));
#22333=CARTESIAN_POINT('Ctrl Pts',(70.0200075220891,23.0360493827148,45.7722265692876));
#22334=CARTESIAN_POINT('Ctrl Pts',(54.7907372267642,22.9258570992293,45.3170284863951));
#22335=CARTESIAN_POINT('Ctrl Pts',(53.7919468056835,21.3912213348628,46.2144683518221));
#22336=CARTESIAN_POINT('Ctrl Pts',(52.7562467146473,17.7832971764642,48.0679863059215));
#22337=CARTESIAN_POINT('Ctrl Pts',(54.5366561274746,12.2550558273829,49.9200347179853));
#22338=CARTESIAN_POINT('Ctrl Pts',(59.4130828744335,8.63727200384955,50.5900930650603));
#22339=CARTESIAN_POINT('Ctrl Pts',(65.5836888418126,8.64389537621032,50.5912639994337));
#22340=CARTESIAN_POINT('Ctrl Pts',(70.4660116067358,12.2531404542804,49.9213697367866));
#22341=CARTESIAN_POINT('Ctrl Pts',(72.2451937624934,17.7836520803225,48.0687233931725));
#22342=CARTESIAN_POINT('Ctrl Pts',(71.2080604594761,21.3912101719866,46.2144748797621));
#22343=CARTESIAN_POINT('Ctrl Pts',(70.2092627732358,22.9258570992293,45.3170284863951));
#22344=CARTESIAN_POINT('Ctrl Pts',(54.2349613371585,22.9441110925392,44.6287642460336));
#22345=CARTESIAN_POINT('Ctrl Pts',(53.1616750836308,21.3176435330343,45.4948761270818));
#22346=CARTESIAN_POINT('Ctrl Pts',(52.0452054104636,17.4934953607748,47.2745378463438));
#22347=CARTESIAN_POINT('Ctrl Pts',(53.9548569140681,11.6579928841,49.0503090096131));
#22348=CARTESIAN_POINT('Ctrl Pts',(59.1876493330094,7.84833229000289,49.7160755075247));
#22349=CARTESIAN_POINT('Ctrl Pts',(65.8088963456918,7.85518686750345,49.7170728023697));
#22350=CARTESIAN_POINT('Ctrl Pts',(71.0479870198883,11.6561154937289,49.0515269255847));
#22351=CARTESIAN_POINT('Ctrl Pts',(72.9563437045815,17.4939164999665,47.2752004277968));
#22352=CARTESIAN_POINT('Ctrl Pts',(71.8383327234084,21.3176317021775,45.4948824271433));
#22353=CARTESIAN_POINT('Ctrl Pts',(70.7650386628414,22.9441110925392,44.6287642460336));
#22354=CARTESIAN_POINT('Ctrl Pts',(53.7050272035642,23.1451548175054,44.3208657108362));
#22355=CARTESIAN_POINT('Ctrl Pts',(52.5348398293169,21.4555874814272,45.2026346040126));
#22356=CARTESIAN_POINT('Ctrl Pts',(51.2465470842867,17.4440228922175,47.0300555365631));
#22357=CARTESIAN_POINT('Ctrl Pts',(53.2226320825593,11.1174259777979,48.8622205971348));
#22358=CARTESIAN_POINT('Ctrl Pts',(58.9168123145029,6.9913313904512,49.5150230715549));
#22359=CARTESIAN_POINT('Ctrl Pts',(66.0802655944533,6.9993885995003,49.5163292093625));
#22360=CARTESIAN_POINT('Ctrl Pts',(71.7804277049591,11.1138898217104,48.8634707307727));
#22361=CARTESIAN_POINT('Ctrl Pts',(73.7550958709857,17.4439130956519,47.0307891232465));
#22362=CARTESIAN_POINT('Ctrl Pts',(72.4651686825769,21.4555751915853,45.2026410179626));
#22363=CARTESIAN_POINT('Ctrl Pts',(71.2949727964358,23.1451548175054,44.3208657108362));
#22364=CARTESIAN_POINT('Ctrl Pts',(53.3864876685926,23.3160685634272,44.2307692307692));
#22365=CARTESIAN_POINT('Ctrl Pts',(52.1577649697301,21.5929471992367,45.1391055895821));
#22366=CARTESIAN_POINT('Ctrl Pts',(50.7654075275861,17.4738130645841,47.0338873948327));
#22367=CARTESIAN_POINT('Ctrl Pts',(52.780390477329,10.8335144477163,48.9382355384849));
#22368=CARTESIAN_POINT('Ctrl Pts',(58.7534376271057,6.49811636507681,49.5800569879468));
#22369=CARTESIAN_POINT('Ctrl Pts',(66.2439626695514,6.50726074921208,49.5814063907908));
#22370=CARTESIAN_POINT('Ctrl Pts',(72.2229368821765,10.828784805706,48.9398470354358));
#22371=CARTESIAN_POINT('Ctrl Pts',(74.2362329569254,17.4733133906627,47.034754231617));
#22372=CARTESIAN_POINT('Ctrl Pts',(72.8422439679473,21.5929346653242,45.1391121967827));
#22373=CARTESIAN_POINT('Ctrl Pts',(71.6135123314074,23.3160685634272,44.2307692307692));
#22374=CARTESIAN_POINT('Ctrl Pts',(69.9640078388351,23.1177228316711,-46.));
#22375=CARTESIAN_POINT('Ctrl Pts',(70.4282880935365,22.448394502084,-46.0000000000001));
#22376=CARTESIAN_POINT('Ctrl Pts',(71.1098490068872,21.4276043550564,-46.));
#22377=CARTESIAN_POINT('Ctrl Pts',(72.1079771651491,20.2176388416739,-46.));
#22378=CARTESIAN_POINT('Ctrl Pts',(72.7378313921175,19.7052440604699,-46.));
#22379=CARTESIAN_POINT('Ctrl Pts',(73.2907028389451,19.5959179422654,-46.));
#22380=CARTESIAN_POINT('Ctrl Pts',(70.150154550487,22.8208715049056,-45.1947514602968));
#22381=CARTESIAN_POINT('Ctrl Pts',(70.7132801788335,22.2671987041132,-45.2933824298082));
#22382=CARTESIAN_POINT('Ctrl Pts',(71.4994124151429,21.3677327932072,-45.5083661587332));
#22383=CARTESIAN_POINT('Ctrl Pts',(72.4178953923351,20.2269070318774,-45.8190912488055));
#22384=CARTESIAN_POINT('Ctrl Pts',(72.9072401408116,19.7267421723513,-45.9597943306481));
#22385=CARTESIAN_POINT('Ctrl Pts',(73.2907028389451,19.5959179422654,-46.));
#22386=CARTESIAN_POINT('Ctrl Pts',(70.862756067458,22.9065587328173,-44.4304270626387));
#22387=CARTESIAN_POINT('Ctrl Pts',(71.3824929671134,22.3609404106397,-44.7176762130643));
#22388=CARTESIAN_POINT('Ctrl Pts',(72.0706374133237,21.4474353285422,-45.1743630927634));
#22389=CARTESIAN_POINT('Ctrl Pts',(72.7587045416073,20.2739035226561,-45.7078285895115));
#22390=CARTESIAN_POINT('Ctrl Pts',(73.0771229289095,19.7538948849925,-45.9327798968234));
#22391=CARTESIAN_POINT('Ctrl Pts',(73.2907028389451,19.5959179422654,-46.));
#22392=CARTESIAN_POINT('Ctrl Pts',(71.6135123331932,23.3160685609229,-44.2307692320894));
#22393=CARTESIAN_POINT('Ctrl Pts',(72.0694661900611,22.6771055141269,-44.5677393482618));
#22394=CARTESIAN_POINT('Ctrl Pts',(72.6451832973973,21.6425621324406,-45.085801261871));
#22395=CARTESIAN_POINT('Ctrl Pts',(73.099528966838,20.3540492246571,-45.6728025929409));
#22396=CARTESIAN_POINT('Ctrl Pts',(73.2470092805887,19.7866035098537,-45.918783509084));
#22397=CARTESIAN_POINT('Ctrl Pts',(73.2907028389451,19.5959179422654,-46.));
#22398=CARTESIAN_POINT('',(69.9640078388351,23.1177228316711,-46.0000000008449));
#22399=CARTESIAN_POINT('Origin',(71.6135123331932,24.2487113033598,-46.000000001373));
#22400=CARTESIAN_POINT('Ctrl Pts',(69.964007837035,23.1177228342965,-46.));
#22401=CARTESIAN_POINT('Ctrl Pts',(70.6700807935817,22.0879417672436,-46.));
#22402=CARTESIAN_POINT('Ctrl Pts',(71.1769284406424,21.365011566508,-46.));
#22403=CARTESIAN_POINT('Ctrl Pts',(71.9178443356484,20.4538645006696,-46.));
#22404=CARTESIAN_POINT('Ctrl Pts',(72.2017412823191,20.1517217214797,-46.));
#22405=CARTESIAN_POINT('Ctrl Pts',(72.6032412874365,19.8400027811803,-46.));
#22406=CARTESIAN_POINT('Ctrl Pts',(72.7445670457876,19.748037119499,-46.0000000000325));
#22407=CARTESIAN_POINT('Ctrl Pts',(72.958561606321,19.656555678685,-46.0000000000325));
#22408=CARTESIAN_POINT('Ctrl Pts',(73.0261035282676,19.6337322451886,-46.));
#22409=CARTESIAN_POINT('Ctrl Pts',(73.1595901689006,19.6038714213038,-46.));
#22410=CARTESIAN_POINT('Ctrl Pts',(73.2248625599985,19.5959179422654,-46.));
#22411=CARTESIAN_POINT('Ctrl Pts',(73.2907028389451,19.5959179422654,-46.));
#22412=CARTESIAN_POINT('Ctrl Pts',(55.0359921629487,23.1177228342728,-46.));
#22413=CARTESIAN_POINT('Ctrl Pts',(55.4577675702659,23.7328665315063,-46.));
#22414=CARTESIAN_POINT('Ctrl Pts',(56.4644460987129,24.8770406742655,-46.));
#22415=CARTESIAN_POINT('Ctrl Pts',(58.4968877073687,26.2505571664569,-46.));
#22416=CARTESIAN_POINT('Ctrl Pts',(61.0767126915491,27.0852062473976,-46.));
#22417=CARTESIAN_POINT('Ctrl Pts',(63.9310735094902,27.0805880901559,-46.));
#22418=CARTESIAN_POINT('Ctrl Pts',(66.5019245727494,26.2505063992629,-46.));
#22419=CARTESIAN_POINT('Ctrl Pts',(68.5371826391601,24.876911244511,-46.));
#22420=CARTESIAN_POINT('Ctrl Pts',(69.5463136462273,23.72691422987,-46.));
#22421=CARTESIAN_POINT('Ctrl Pts',(69.9640078384976,23.1177228321634,-46.));
#22422=CARTESIAN_POINT('Ctrl Pts',(54.9799924778935,23.036049382692,-45.7722265692886));
#22423=CARTESIAN_POINT('Ctrl Pts',(55.429815478711,23.6267219749649,-45.7450333341526));
#22424=CARTESIAN_POINT('Ctrl Pts',(56.4988342870035,24.6938856008765,-45.7247629982864));
#22425=CARTESIAN_POINT('Ctrl Pts',(58.5542027836181,25.9190899660437,-45.7850931685235));
#22426=CARTESIAN_POINT('Ctrl Pts',(61.0913426462871,26.65821922096,-45.8854831073846));
#22427=CARTESIAN_POINT('Ctrl Pts',(63.9157961167037,26.6541165160517,-45.8838942577118));
#22428=CARTESIAN_POINT('Ctrl Pts',(66.4440587647699,25.9184853590342,-45.7844551748528));
#22429=CARTESIAN_POINT('Ctrl Pts',(68.5030877198132,24.6937964378016,-45.7240503148626));
#22430=CARTESIAN_POINT('Ctrl Pts',(69.5745371341163,23.6210064625856,-45.7452964634328));
#22431=CARTESIAN_POINT('Ctrl Pts',(70.0200075236488,23.0360493806665,-45.772226569382));
#22432=CARTESIAN_POINT('Ctrl Pts',(54.7907802349192,22.9256684193329,-45.3167264994694));
#22433=CARTESIAN_POINT('Ctrl Pts',(55.2841708894856,23.4853279772414,-45.2164752999044));
#22434=CARTESIAN_POINT('Ctrl Pts',(56.4679989024545,24.4367980894975,-45.0977591258001));
#22435=CARTESIAN_POINT('Ctrl Pts',(58.6119105347406,25.3836007202491,-45.1590251424147));
#22436=CARTESIAN_POINT('Ctrl Pts',(61.112821395526,25.8840372741794,-45.3603121455667));
#22437=CARTESIAN_POINT('Ctrl Pts',(63.8938482330649,25.8822538891794,-45.3568243041171));
#22438=CARTESIAN_POINT('Ctrl Pts',(66.3853316497856,25.3831132440572,-45.1570554139588));
#22439=CARTESIAN_POINT('Ctrl Pts',(68.5344243155597,24.4373495148053,-45.0958874813595));
#22440=CARTESIAN_POINT('Ctrl Pts',(69.7206032961255,23.479912555677,-45.2174453583454));
#22441=CARTESIAN_POINT('Ctrl Pts',(70.2092197667725,22.9256684174138,-45.3167264998131));
#22442=CARTESIAN_POINT('Ctrl Pts',(54.3540307949898,22.940312374942,-44.7764305165133));
#22443=CARTESIAN_POINT('Ctrl Pts',(54.8725241139022,23.5168125343872,-44.5569401518282));
#22444=CARTESIAN_POINT('Ctrl Pts',(56.1694841702895,24.4531474854901,-44.2164314277651));
#22445=CARTESIAN_POINT('Ctrl Pts',(58.5098618481284,25.2243797451509,-44.0490074515783));
#22446=CARTESIAN_POINT('Ctrl Pts',(61.1059304240575,25.4905041608905,-44.1402636454315));
#22447=CARTESIAN_POINT('Ctrl Pts',(63.901828202477,25.4917212441726,-44.1370682351324));
#22448=CARTESIAN_POINT('Ctrl Pts',(66.4865076249529,25.2254109591687,-44.0467524245259));
#22449=CARTESIAN_POINT('Ctrl Pts',(68.8333479287006,24.4549911624279,-44.2145400319697));
#22450=CARTESIAN_POINT('Ctrl Pts',(70.132492972152,23.5112341585224,-44.5590640016221));
#22451=CARTESIAN_POINT('Ctrl Pts',(70.6459692067881,22.9403123729652,-44.776430517266));
#22452=CARTESIAN_POINT('Ctrl Pts',(53.8642397535411,23.0841835154313,-44.4122888532322));
#22453=CARTESIAN_POINT('Ctrl Pts',(54.3852644864179,23.7210088220369,-44.0947795647735));
#22454=CARTESIAN_POINT('Ctrl Pts',(55.7542433739063,24.7573036807876,-43.5521310136212));
#22455=CARTESIAN_POINT('Ctrl Pts',(58.3038539355888,25.5714931127472,-43.1253852425921));
#22456=CARTESIAN_POINT('Ctrl Pts',(61.0735166591671,25.7929641498958,-43.0408658934962));
#22457=CARTESIAN_POINT('Ctrl Pts',(63.9360342309663,25.7953039701295,-43.0390901749241));
#22458=CARTESIAN_POINT('Ctrl Pts',(66.692119856051,25.5734728698309,-43.1234808632927));
#22459=CARTESIAN_POINT('Ctrl Pts',(69.2487599668007,24.7597018881128,-43.5508755354234));
#22460=CARTESIAN_POINT('Ctrl Pts',(70.619777094379,23.714846723268,-44.097851872979));
#22461=CARTESIAN_POINT('Ctrl Pts',(71.1357602482455,23.0841835132476,-44.4122888543209));
#22462=CARTESIAN_POINT('Ctrl Pts',(53.5457574360584,23.2306116904395,-44.2758174708167));
#22463=CARTESIAN_POINT('Ctrl Pts',(54.0627762662708,23.9223005711454,-43.9129480259072));
#22464=CARTESIAN_POINT('Ctrl Pts',(55.4662284705153,25.0651176112046,-43.2722290901921));
#22465=CARTESIAN_POINT('Ctrl Pts',(58.1486595615419,25.9902484809716,-42.7163490041473));
#22466=CARTESIAN_POINT('Ctrl Pts',(61.0464675813894,26.2644288113384,-42.547000973267));
#22467=CARTESIAN_POINT('Ctrl Pts',(63.9643601544157,26.2666452488003,-42.5458771037084));
#22468=CARTESIAN_POINT('Ctrl Pts',(66.847174393407,25.9923497630692,-42.7145138052446));
#22469=CARTESIAN_POINT('Ctrl Pts',(69.5368351511896,25.0674401569483,-43.2712998655934));
#22470=CARTESIAN_POINT('Ctrl Pts',(70.9422265523446,23.9156075971566,-43.9164592516275));
#22471=CARTESIAN_POINT('Ctrl Pts',(71.4542425657144,23.2306116880677,-44.2758174720609));
#22472=CARTESIAN_POINT('Ctrl Pts',(53.3864876685727,23.3160685633993,-44.2307692307839));
#22473=CARTESIAN_POINT('Ctrl Pts',(53.9014731106537,24.038267655457,-43.8500649418989));
#22474=CARTESIAN_POINT('Ctrl Pts',(55.3220849100951,25.2411372376895,-43.1704876695772));
#22475=CARTESIAN_POINT('Ctrl Pts',(58.0708968314258,26.2337622543912,-42.5667104493236));
#22476=CARTESIAN_POINT('Ctrl Pts',(61.0328912216257,26.5456758334602,-42.3710278989254));
#22477=CARTESIAN_POINT('Ctrl Pts',(63.9785719433368,26.5476372801886,-42.3700397756168));
#22478=CARTESIAN_POINT('Ctrl Pts',(66.9248798545188,26.2358932678842,-42.5648089417427));
#22479=CARTESIAN_POINT('Ctrl Pts',(69.681000122088,25.243380770632,-43.1696388054261));
#22480=CARTESIAN_POINT('Ctrl Pts',(71.1035100323559,24.0312794561666,-43.8537487425401));
#22481=CARTESIAN_POINT('Ctrl Pts',(71.6135123331932,23.3160685609229,-44.2307692320894));
#22482=CARTESIAN_POINT('',(55.0359921629504,23.1177228342752,-46.0000000000069));
#22483=CARTESIAN_POINT('Origin',(53.3864876685947,24.2487113059674,-45.9999999999984));
#22484=CARTESIAN_POINT('Origin',(62.5,18.,-46.));
#22485=CARTESIAN_POINT('Ctrl Pts',(51.7092971610549,19.5959179422654,-46.));
#22486=CARTESIAN_POINT('Ctrl Pts',(52.2620653939839,19.7051356050392,-46.));
#22487=CARTESIAN_POINT('Ctrl Pts',(52.8920949226161,20.2177543439005,-46.));
#22488=CARTESIAN_POINT('Ctrl Pts',(53.8897778317011,21.4271096929168,-45.9999999999999));
#22489=CARTESIAN_POINT('Ctrl Pts',(54.5713813881105,22.4479061064219,-46.0000000000001));
#22490=CARTESIAN_POINT('Ctrl Pts',(55.0359921629652,23.1177228342968,-46.));
#22491=CARTESIAN_POINT('Ctrl Pts',(51.7092971610548,19.5959179422654,-46.));
#22492=CARTESIAN_POINT('Ctrl Pts',(52.0926675666913,19.7266394067263,-45.9598226817129));
#22493=CARTESIAN_POINT('Ctrl Pts',(52.5821841468467,20.2270134514137,-45.819062250804));
#22494=CARTESIAN_POINT('Ctrl Pts',(53.5002246591862,21.3672689127023,-45.5084940953287));
#22495=CARTESIAN_POINT('Ctrl Pts',(54.2863195908853,22.2667867790925,-45.2934650574444));
#22496=CARTESIAN_POINT('Ctrl Pts',(54.849845451707,22.8208715070777,-45.194751459911));
#22497=CARTESIAN_POINT('Ctrl Pts',(51.709297161055,19.5959179422654,-46.));
#22498=CARTESIAN_POINT('Ctrl Pts',(51.9228095515637,19.753788288119,-45.9328286977184));
#22499=CARTESIAN_POINT('Ctrl Pts',(52.2413619039012,20.2740130336108,-45.7077763242479));
#22500=CARTESIAN_POINT('Ctrl Pts',(52.9290812390771,21.4469571597183,-45.1745842010763));
#22501=CARTESIAN_POINT('Ctrl Pts',(53.6171415340253,22.3605295352944,-44.7178900299161));
#22502=CARTESIAN_POINT('Ctrl Pts',(54.1372439345722,22.9065587349562,-44.4304270615132));
#22503=CARTESIAN_POINT('Ctrl Pts',(51.7092971610549,19.5959179422654,-46.));
#22504=CARTESIAN_POINT('Ctrl Pts',(51.7529482282219,19.7864858334401,-45.9188374584652));
#22505=CARTESIAN_POINT('Ctrl Pts',(51.9005239862315,20.3541704296053,-45.6727447106325));
#22506=CARTESIAN_POINT('Ctrl Pts',(52.3546179283007,21.6420362564594,-45.0860447448006));
#22507=CARTESIAN_POINT('Ctrl Pts',(52.930215177034,22.6766294615115,-44.5679874350866));
#22508=CARTESIAN_POINT('Ctrl Pts',(53.3864876685928,23.3160685634274,-44.2307692307691));
#22509=CARTESIAN_POINT('Ctrl Pts',(51.7092971610549,19.5959179422654,-46.));
#22510=CARTESIAN_POINT('Ctrl Pts',(52.2620653939839,19.7051356050392,-46.));
#22511=CARTESIAN_POINT('Ctrl Pts',(52.4720752368613,19.876008517993,-46.));
#22512=CARTESIAN_POINT('Ctrl Pts',(52.659590508736,20.0475121432486,-46.));
#22513=CARTESIAN_POINT('Ctrl Pts',(53.0346210524853,20.39051939376,-46.));
#22514=CARTESIAN_POINT('Ctrl Pts',(53.3196733122239,20.7360494934789,-46.));
#22515=CARTESIAN_POINT('Ctrl Pts',(53.5854418805396,21.0798247170144,-46.));
#22516=CARTESIAN_POINT('Ctrl Pts',(54.1169790171708,21.7673751640851,-46.));
#22517=CARTESIAN_POINT('Ctrl Pts',(54.5713813881103,22.4479061064217,-46.0000000000001));
#22518=CARTESIAN_POINT('Ctrl Pts',(55.035992162965,23.1177228342965,-46.));
#22519=CARTESIAN_POINT('Ctrl Pts',(69.964007837035,23.1177228342965,-46.));
#22520=CARTESIAN_POINT('Ctrl Pts',(70.9703372872347,21.6500288723272,-46.9446698131655));
#22521=CARTESIAN_POINT('Ctrl Pts',(72.1183944604502,18.1446538308373,-48.9200122557279));
#22522=CARTESIAN_POINT('Ctrl Pts',(70.4543334202127,12.483202392177,-50.8920744141013));
#22523=CARTESIAN_POINT('Ctrl Pts',(65.5691776348049,8.79342862675378,-51.5637399768993));
#22524=CARTESIAN_POINT('Ctrl Pts',(59.4328684025022,8.80019559553396,-51.5641637407931));
#22525=CARTESIAN_POINT('Ctrl Pts',(54.5371355691,12.4816854912179,-50.8976114017526));
#22526=CARTESIAN_POINT('Ctrl Pts',(52.8878093794935,18.1409814039487,-48.9160426988189));
#22527=CARTESIAN_POINT('Ctrl Pts',(54.0296553927672,21.650018196383,-46.944676684654));
#22528=CARTESIAN_POINT('Ctrl Pts',(55.035992162965,23.1177228342965,-46.));
#22529=CARTESIAN_POINT('Ctrl Pts',(70.0200075220892,23.0360493827148,-45.7722265692876));
#22530=CARTESIAN_POINT('Ctrl Pts',(71.0163635385786,21.548387511723,-46.7011217010093));
#22531=CARTESIAN_POINT('Ctrl Pts',(72.1116609454533,18.0207073641069,-48.6369541642022));
#22532=CARTESIAN_POINT('Ctrl Pts',(70.4070372012184,12.4400174548645,-50.5666834109832));
#22533=CARTESIAN_POINT('Ctrl Pts',(65.5574758632647,8.79647831783238,-51.238894394837));
#22534=CARTESIAN_POINT('Ctrl Pts',(59.444982641667,8.80290739556665,-51.2393092746466));
#22535=CARTESIAN_POINT('Ctrl Pts',(54.5854421071155,12.438947874978,-50.5718180574722));
#22536=CARTESIAN_POINT('Ctrl Pts',(52.8932465944024,18.0179605889219,-48.6332915172475));
#22537=CARTESIAN_POINT('Ctrl Pts',(53.9836292139696,21.5483766905331,-46.7011284577535));
#22538=CARTESIAN_POINT('Ctrl Pts',(54.9799924779108,23.0360493827148,-45.7722265692876));
#22539=CARTESIAN_POINT('Ctrl Pts',(70.2092627732358,22.9258570992293,-45.3170284863951));
#22540=CARTESIAN_POINT('Ctrl Pts',(71.2080531943165,21.3912213348628,-46.2144683518222));
#22541=CARTESIAN_POINT('Ctrl Pts',(72.2485073332692,17.7848938426267,-48.0716979134992));
#22542=CARTESIAN_POINT('Ctrl Pts',(70.4595522749644,12.2538636517655,-49.9171964156177));
#22543=CARTESIAN_POINT('Ctrl Pts',(65.5872688285877,8.63757133840816,-50.5904626682655));
#22544=CARTESIAN_POINT('Ctrl Pts',(59.4158247717921,8.64370707313489,-50.5908806139701));
#22545=CARTESIAN_POINT('Ctrl Pts',(54.5341291044486,12.2532305473249,-49.9215007698885));
#22546=CARTESIAN_POINT('Ctrl Pts',(52.7547119853049,17.7836087469459,-48.0686452362413));
#22547=CARTESIAN_POINT('Ctrl Pts',(53.7919395405239,21.3912101719867,-46.2144748797621));
#22548=CARTESIAN_POINT('Ctrl Pts',(54.7907372267642,22.9258570992293,-45.3170284863951));
#22549=CARTESIAN_POINT('Ctrl Pts',(70.7650386628415,22.9441110925393,-44.6287642460337));
#22550=CARTESIAN_POINT('Ctrl Pts',(71.8383249163693,21.3176435330343,-45.4948761270819));
#22551=CARTESIAN_POINT('Ctrl Pts',(72.9598945847606,17.4948749234169,-47.277728446391));
#22552=CARTESIAN_POINT('Ctrl Pts',(71.0410755502145,11.6569613647031,-49.047848196163));
#22553=CARTESIAN_POINT('Ctrl Pts',(65.8127297003932,7.84860393154229,-49.7164030171663));
#22554=CARTESIAN_POINT('Ctrl Pts',(59.1905815389834,7.85502151184498,-49.7167388747517));
#22555=CARTESIAN_POINT('Ctrl Pts',(53.9521643544241,11.6561965293243,-49.0516422890679));
#22556=CARTESIAN_POINT('Ctrl Pts',(52.0435550568373,17.4938780779608,-47.2751321156197));
#22557=CARTESIAN_POINT('Ctrl Pts',(53.1616672765916,21.3176317021776,-45.4948824271434));
#22558=CARTESIAN_POINT('Ctrl Pts',(54.2349613371585,22.9441110925393,-44.6287642460337));
#22559=CARTESIAN_POINT('Ctrl Pts',(71.2949727964358,23.1451548175053,-44.3208657108362));
#22560=CARTESIAN_POINT('Ctrl Pts',(72.4651601706831,21.4555874814272,-45.2026346040127));
#22561=CARTESIAN_POINT('Ctrl Pts',(73.7611756319396,17.4466520281733,-47.0338832915689));
#22562=CARTESIAN_POINT('Ctrl Pts',(71.7712823336433,11.1154328342175,-48.8593967521573));
#22563=CARTESIAN_POINT('Ctrl Pts',(66.0838726210504,6.99188921257162,-49.5153685816591));
#22564=CARTESIAN_POINT('Ctrl Pts',(58.9189313583151,6.99906255642572,-49.5159529203514));
#22565=CARTESIAN_POINT('Ctrl Pts',(53.2198273601607,11.1140544776842,-48.8635955038756));
#22566=CARTESIAN_POINT('Ctrl Pts',(51.24474414428,17.443836399062,-47.0307131526209));
#22567=CARTESIAN_POINT('Ctrl Pts',(52.5348313174231,21.4555751915854,-45.2026410179625));
#22568=CARTESIAN_POINT('Ctrl Pts',(53.7050272035642,23.1451548175053,-44.3208657108362));
#22569=CARTESIAN_POINT('Ctrl Pts',(71.6135123314074,23.3160685634272,-44.2307692307692));
#22570=CARTESIAN_POINT('Ctrl Pts',(72.84223503027,21.5929471992366,-45.1391055895822));
#22571=CARTESIAN_POINT('Ctrl Pts',(74.2440064959087,17.4775207002499,-47.0384733228152));
#22572=CARTESIAN_POINT('Ctrl Pts',(72.2121971594862,10.8307890388393,-48.9346869366359));
#22573=CARTESIAN_POINT('Ctrl Pts',(66.2474489353142,6.49887232528998,-49.580519208557));
#22574=CARTESIAN_POINT('Ctrl Pts',(58.7550492649336,6.50681697095731,-49.5809266738395));
#22575=CARTESIAN_POINT('Ctrl Pts',(52.7773865235972,10.8290081468293,-48.9400109632237));
#22576=CARTESIAN_POINT('Ctrl Pts',(50.7635683583871,17.4732091493448,-47.0346564411719));
#22577=CARTESIAN_POINT('Ctrl Pts',(52.1577560320527,21.5929346653243,-45.1391121967827));
#22578=CARTESIAN_POINT('Ctrl Pts',(53.3864876685926,23.3160685634272,-44.2307692307692));
#22579=CARTESIAN_POINT('',(53.4480382353792,18.0006404973954,-48.7869877464486));
#22580=CARTESIAN_POINT('Ctrl Pts',(69.9640078386373,23.1177228319597,-46.0000000015041));
#22581=CARTESIAN_POINT('Ctrl Pts',(70.970337287844,21.6500288704668,-46.9446698142138));
#22582=CARTESIAN_POINT('Ctrl Pts',(72.1183944601558,18.1446538298357,-48.9200122560767));
#22583=CARTESIAN_POINT('Ctrl Pts',(70.4543334202127,12.483202392177,-50.8920744141013));
#22584=CARTESIAN_POINT('Ctrl Pts',(65.5691776348049,8.79342862675378,-51.5637399768993));
#22585=CARTESIAN_POINT('Ctrl Pts',(59.4328684025022,8.80019559553396,-51.5641637407931));
#22586=CARTESIAN_POINT('Ctrl Pts',(54.5593513886519,12.4649796541169,-50.9006360779329));
#22587=CARTESIAN_POINT('Ctrl Pts',(53.4526536488011,16.20324910153,-49.5945088774883));
#22588=CARTESIAN_POINT('Ctrl Pts',(53.4480382353792,18.0006404973954,-48.7869877464486));
#22589=CARTESIAN_POINT('Ctrl Pts',(53.4480382353792,18.0006404973954,-48.7869877464486));
#22590=CARTESIAN_POINT('Ctrl Pts',(53.4479745368625,18.025446761822,-48.7758429380598));
#22591=CARTESIAN_POINT('Ctrl Pts',(53.450960195781,19.8716148791025,-47.9437781664976));
#22592=CARTESIAN_POINT('Ctrl Pts',(54.0296553927672,21.650018196383,-46.944676684654));
#22593=CARTESIAN_POINT('Ctrl Pts',(55.035992162965,23.1177228342965,-46.));
#22594=CARTESIAN_POINT('Origin',(62.5,18.,-64.));
#22595=CARTESIAN_POINT('',(53.45,18.,-64.));
#22596=CARTESIAN_POINT('Origin',(99.8,45.,-45.));
#22597=CARTESIAN_POINT('Origin',(99.8,-45.,45.));
#22598=CARTESIAN_POINT('Origin',(99.8,45.,45.));
#22599=CARTESIAN_POINT('Origin',(99.8,-45.,-45.));
#22600=CARTESIAN_POINT('Origin',(-4.8,0.,0.));
#22601=CARTESIAN_POINT('',(-9.5,-23.525,-2.88098159499415E-15));
#22602=CARTESIAN_POINT('Origin',(-9.5,0.,0.));
#22603=CARTESIAN_POINT('',(0.,-23.525,-2.88098159499415E-15));
#22604=CARTESIAN_POINT('',(-4.8,-23.525,-2.88098159499415E-15));
#22605=CARTESIAN_POINT('Origin',(0.,0.,0.));
#22606=CARTESIAN_POINT('Origin',(0.,27.505,0.));
#22607=CARTESIAN_POINT('',(-1.11022302462516E-15,-27.505,-3.36839102105479E-15));
#22608=CARTESIAN_POINT('Origin',(0.,0.,0.));
#22609=CARTESIAN_POINT('Origin',(6.99999999999999,0.,0.));
#22610=CARTESIAN_POINT('',(14.,-27.505,-3.36839102105479E-15));
#22611=CARTESIAN_POINT('',(6.99999999999999,-27.505,-3.36839102105479E-15));
#22612=CARTESIAN_POINT('Origin',(14.,0.,0.));
#22613=CARTESIAN_POINT('Origin',(14.,26.,0.));
#22614=CARTESIAN_POINT('',(14.,-26.,-3.18408167778312E-15));
#22615=CARTESIAN_POINT('Origin',(14.,0.,0.));
#22616=CARTESIAN_POINT('Origin',(15.,0.,0.));
#22617=CARTESIAN_POINT('',(16.,-26.,-3.18408167778312E-15));
#22618=CARTESIAN_POINT('',(15.,-26.,-3.18408167778312E-15));
#22619=CARTESIAN_POINT('Origin',(16.,0.,0.));
#22620=CARTESIAN_POINT('Origin',(16.,50.,0.));
#22621=CARTESIAN_POINT('Origin',(-9.5,50.3,0.));
#22622=CARTESIAN_POINT('Origin',(16.,-32.,32.));
#22623=CARTESIAN_POINT('Origin',(16.,-32.,-32.));
#22624=CARTESIAN_POINT('Origin',(16.,0.,0.));
#22625=CARTESIAN_POINT('Origin',(16.,0.,0.));
#38475=UNCERTAINTY_MEASURE_WITH_UNIT(LENGTH_MEASURE(0.01),#38508,
'DISTANCE_ACCURACY_VALUE',
'Maximum model space distance between geometric entities at asserted c
onnectivities');
#38490=UNCERTAINTY_MEASURE_WITH_UNIT(LENGTH_MEASURE(0.01),#38508,
'DISTANCE_ACCURACY_VALUE',
'Maximum model space distance between geometric entities at asserted c
onnectivities');
#38492=(
GEOMETRIC_REPRESENTATION_CONTEXT(3)
GLOBAL_UNCERTAINTY_ASSIGNED_CONTEXT((#38475))
GLOBAL_UNIT_ASSIGNED_CONTEXT((#38508,#38510,#38511))
REPRESENTATION_CONTEXT('','3D')
);
#38507=(
GEOMETRIC_REPRESENTATION_CONTEXT(3)
GLOBAL_UNCERTAINTY_ASSIGNED_CONTEXT((#38490))
GLOBAL_UNIT_ASSIGNED_CONTEXT((#38508,#38510,#38511))
REPRESENTATION_CONTEXT('','3D')
);
#38508=(
LENGTH_UNIT()
NAMED_UNIT(*)
SI_UNIT(.MILLI.,.METRE.)
);
#38510=(
NAMED_UNIT(*)
PLANE_ANGLE_UNIT()
SI_UNIT($,.RADIAN.)
);
#38511=(
NAMED_UNIT(*)
SI_UNIT($,.STERADIAN.)
SOLID_ANGLE_UNIT()
);
#38513=SHAPE_DEFINITION_REPRESENTATION(#38529,#38575);
#38529=PRODUCT_DEFINITION_SHAPE('',$,#38592);
#38575=SHAPE_REPRESENTATION('',(#15253),#38492);
#38590=PRODUCT_DEFINITION_CONTEXT('part definition',#38640,'design');
#38592=PRODUCT_DEFINITION('2026-10-26-01-10-34-522',
'01_Housing_SAE_B_Flange',#38608,#38590);
#38608=PRODUCT_DEFINITION_FORMATION('',$,#38643);
#38640=APPLICATION_CONTEXT(
'Core Data for Automotive Mechanical Design Process');
#38641=PRODUCT_CONTEXT('part definition',#38640,'mechanical');
#38643=PRODUCT('2026-10-26-01-10-34-522','01_Housing_SAE_B_Flange',$,(#38641));
#38693=COLOUR_RGB('Dark Blue',0.08,0.2,0.34);
#38694=FILL_AREA_STYLE_COLOUR('',#38693);
#38695=FILL_AREA_STYLE('',(#38694));
#38696=SURFACE_STYLE_FILL_AREA(#38695);
#38697=SURFACE_SIDE_STYLE('',(#38696));
#38698=SURFACE_STYLE_USAGE(.BOTH.,#38697);
#38699=PRESENTATION_STYLE_ASSIGNMENT((#38698));
ENDSEC;
END-ISO-10303-21;
